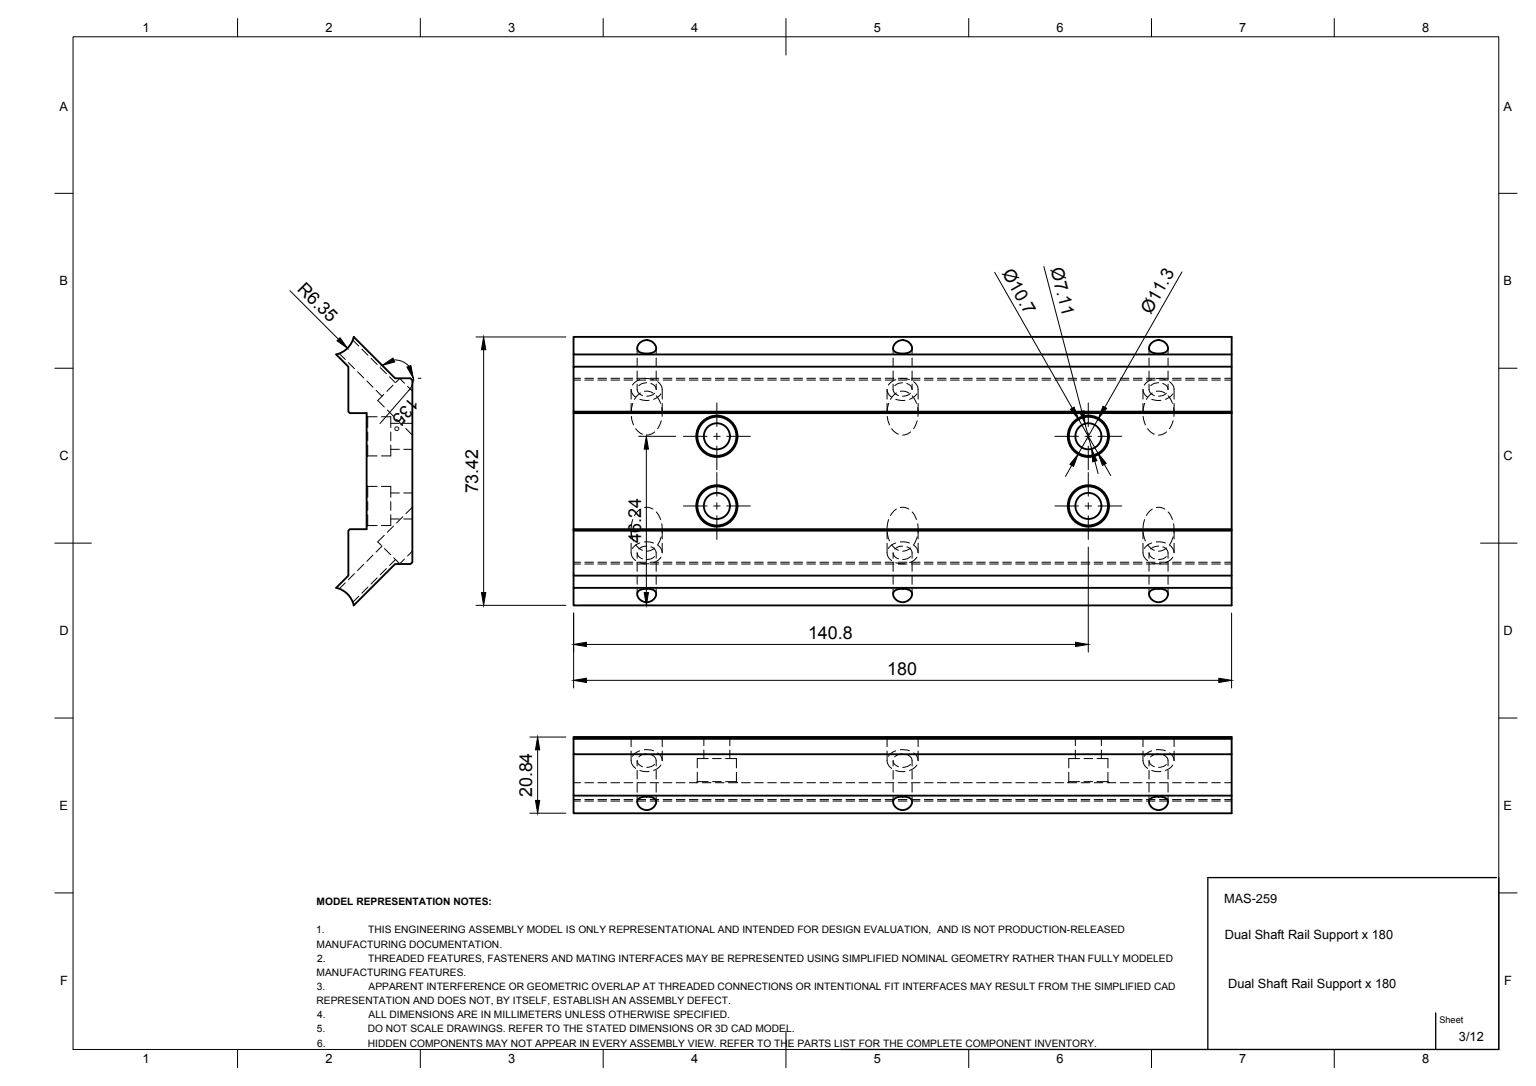
ISO-10303-21;
HEADER;
/* Generated by software containing ST-Developer
 * from STEP Tools, Inc. (www.steptools.com) 
 */

FILE_DESCRIPTION(
/* description */ (''),
/* implementation_level */ '2;1');

FILE_NAME(
/* name */ 'Dual Shaft Rail Support x 180.step',
/* time_stamp */ '2026-10-15T13:30:17-07:00',
/* author */ (''),
/* organization */ (''),
/* preprocessor_version */ 'ST-DEVELOPER v20.2',
/* originating_system */ 'Autodesk Translation Framework v15.15.0.0',
/* authorisation */ '');

FILE_SCHEMA (('AUTOMOTIVE_DESIGN { 1 0 10303 214 3 1 1 }'));
ENDSEC;

DATA;
#10=MECHANICAL_DESIGN_GEOMETRIC_PRESENTATION_REPRESENTATION('',(#1033),#71795);
#1013=SHAPE_REPRESENTATION_RELATIONSHIP('SRR','None',#72017,#1023);
#1023=ADVANCED_BREP_SHAPE_REPRESENTATION('',(#1043),#71785);
#1033=STYLED_ITEM('',(#72076),#1043);
#1043=MANIFOLD_SOLID_BREP('Body1',#13635);
#1053=CONICAL_SURFACE('',#13794,5.5,0.785398163397437);
#1054=CONICAL_SURFACE('',#13803,5.5,0.785398163397452);
#1055=CONICAL_SURFACE('',#13807,5.5,0.785398163397452);
#1056=CONICAL_SURFACE('',#13811,5.5,0.785398163397437);
#1103=B_SPLINE_CURVE_WITH_KNOTS('',3,(#18543,#18544,#18545,#18546,#18547,
#18548,#18549,#18550,#18551,#18552,#18553,#18554,#18555,#18556,#18557,#18558,
#18559,#18560),.UNSPECIFIED.,.F.,.F.,(4,2,2,2,2,2,2,2,4),(-1.58749465662543,
-1.48822066272646,-1.3889466688275,-1.28978383064828,-1.19062099246907,
-1.09145815428986,-0.992295316110649,-0.893021322211684,-0.793747328312718),
 .UNSPECIFIED.);
#1104=B_SPLINE_CURVE_WITH_KNOTS('',3,(#18561,#18562,#18563,#18564,#18565,
#18566,#18567,#18568,#18569,#18570,#18571,#18572,#18573,#18574,#18575,#18576,
#18577,#18578),.UNSPECIFIED.,.F.,.F.,(4,2,2,2,2,2,2,2,4),(-0.793747328312718,
-0.694473334413751,-0.595199340514785,-0.496036502335572,-0.39687366415636,
-0.297710825977147,-0.198547987797934,-0.0992739938989668,0.),
 .UNSPECIFIED.);
#1105=B_SPLINE_CURVE_WITH_KNOTS('',3,(#18592,#18593,#18594,#18595,#18596,
#18597,#18598,#18599,#18600,#18601,#18602,#18603,#18604,#18605,#18606,#18607,
#18608,#18609),.UNSPECIFIED.,.F.,.F.,(4,2,2,2,2,2,2,2,4),(-1.58749465662543,
-1.48822066272646,-1.38894666882749,-1.28978383064828,-1.19062099246907,
-1.09145815428986,-0.992295316110645,-0.893021322211679,-0.793747328312713),
 .UNSPECIFIED.);
#1106=B_SPLINE_CURVE_WITH_KNOTS('',3,(#18610,#18611,#18612,#18613,#18614,
#18615,#18616,#18617,#18618,#18619,#18620,#18621,#18622,#18623,#18624,#18625,
#18626,#18627),.UNSPECIFIED.,.F.,.F.,(4,2,2,2,2,2,2,2,4),(-0.793747328312713,
-0.694473334413747,-0.595199340514781,-0.496036502335569,-0.396873664156357,
-0.297710825977144,-0.198547987797932,-0.0992739938989662,0.),
 .UNSPECIFIED.);
#1107=B_SPLINE_CURVE_WITH_KNOTS('',3,(#18641,#18642,#18643,#18644,#18645,
#18646,#18647,#18648,#18649,#18650,#18651,#18652,#18653,#18654,#18655,#18656,
#18657,#18658),.UNSPECIFIED.,.F.,.F.,(4,2,2,2,2,2,2,2,4),(-1.58749465662542,
-1.48822066272646,-1.38894666882749,-1.28978383064828,-1.19062099246907,
-1.09145815428986,-0.992295316110644,-0.893021322211679,-0.793747328312713),
 .UNSPECIFIED.);
#1108=B_SPLINE_CURVE_WITH_KNOTS('',3,(#18659,#18660,#18661,#18662,#18663,
#18664,#18665,#18666,#18667,#18668,#18669,#18670,#18671,#18672,#18673,#18674,
#18675,#18676),.UNSPECIFIED.,.F.,.F.,(4,2,2,2,2,2,2,2,4),(-0.793747328312713,
-0.694473334413747,-0.595199340514781,-0.496036502335569,-0.396873664156357,
-0.297710825977144,-0.198547987797932,-0.099273993898966,0.),
 .UNSPECIFIED.);
#1109=B_SPLINE_CURVE_WITH_KNOTS('',3,(#18690,#18691,#18692,#18693,#18694,
#18695,#18696,#18697,#18698,#18699,#18700,#18701,#18702,#18703,#18704,#18705,
#18706,#18707),.UNSPECIFIED.,.F.,.F.,(4,2,2,2,2,2,2,2,4),(-1.58749465662543,
-1.48822066272646,-1.3889466688275,-1.28978383064828,-1.19062099246907,
-1.09145815428986,-0.992295316110649,-0.893021322211684,-0.793747328312718),
 .UNSPECIFIED.);
#1110=B_SPLINE_CURVE_WITH_KNOTS('',3,(#18708,#18709,#18710,#18711,#18712,
#18713,#18714,#18715,#18716,#18717,#18718,#18719,#18720,#18721,#18722,#18723,
#18724,#18725),.UNSPECIFIED.,.F.,.F.,(4,2,2,2,2,2,2,2,4),(-0.793747328312718,
-0.694473334413751,-0.595199340514785,-0.496036502335572,-0.396873664156359,
-0.297710825977146,-0.198547987797934,-0.0992739938989669,0.),
 .UNSPECIFIED.);
#1111=B_SPLINE_CURVE_WITH_KNOTS('',3,(#18739,#18740,#18741,#18742,#18743,
#18744,#18745,#18746,#18747,#18748,#18749,#18750,#18751,#18752,#18753,#18754,
#18755,#18756),.UNSPECIFIED.,.F.,.F.,(4,2,2,2,2,2,2,2,4),(-1.58749465662543,
-1.48822066272646,-1.38894666882749,-1.28978383064828,-1.19062099246907,
-1.09145815428986,-0.992295316110645,-0.893021322211679,-0.793747328312713),
 .UNSPECIFIED.);
#1112=B_SPLINE_CURVE_WITH_KNOTS('',3,(#18757,#18758,#18759,#18760,#18761,
#18762,#18763,#18764,#18765,#18766,#18767,#18768,#18769,#18770,#18771,#18772,
#18773,#18774),.UNSPECIFIED.,.F.,.F.,(4,2,2,2,2,2,2,2,4),(-0.793747328312713,
-0.694473334413747,-0.595199340514781,-0.496036502335568,-0.396873664156356,
-0.297710825977144,-0.198547987797932,-0.099273993898966,0.),
 .UNSPECIFIED.);
#1113=B_SPLINE_CURVE_WITH_KNOTS('',3,(#18788,#18789,#18790,#18791,#18792,
#18793,#18794,#18795,#18796,#18797,#18798,#18799,#18800,#18801,#18802,#18803,
#18804,#18805),.UNSPECIFIED.,.F.,.F.,(4,2,2,2,2,2,2,2,4),(-1.58749465662543,
-1.48822066272646,-1.38894666882749,-1.28978383064828,-1.19062099246907,
-1.09145815428986,-0.992295316110644,-0.893021322211679,-0.793747328312713),
 .UNSPECIFIED.);
#1114=B_SPLINE_CURVE_WITH_KNOTS('',3,(#18806,#18807,#18808,#18809,#18810,
#18811,#18812,#18813,#18814,#18815,#18816,#18817,#18818,#18819,#18820,#18821,
#18822,#18823),.UNSPECIFIED.,.F.,.F.,(4,2,2,2,2,2,2,2,4),(-0.793747328312713,
-0.694473334413747,-0.595199340514781,-0.496036502335569,-0.396873664156356,
-0.297710825977144,-0.198547987797932,-0.0992739938989659,0.),
 .UNSPECIFIED.);
#1484=FACE_BOUND('',#2677,.T.);
#1485=FACE_BOUND('',#2681,.T.);
#1486=FACE_BOUND('',#2685,.T.);
#1487=FACE_BOUND('',#2689,.T.);
#1488=FACE_BOUND('',#2693,.T.);
#1489=FACE_BOUND('',#2697,.T.);
#1490=FACE_BOUND('',#2701,.T.);
#1491=FACE_BOUND('',#2702,.T.);
#1492=FACE_BOUND('',#2703,.T.);
#1493=FACE_BOUND('',#2704,.T.);
#1494=FACE_BOUND('',#2713,.T.);
#1495=FACE_BOUND('',#2715,.T.);
#1496=FACE_BOUND('',#2717,.T.);
#1497=FACE_BOUND('',#2719,.T.);
#1498=FACE_BOUND('',#2731,.T.);
#1499=FACE_BOUND('',#2732,.T.);
#1500=FACE_BOUND('',#2733,.T.);
#1501=FACE_BOUND('',#2734,.T.);
#1502=FACE_BOUND('',#2735,.T.);
#1503=FACE_BOUND('',#2736,.T.);
#1504=FACE_BOUND('',#2737,.T.);
#1505=FACE_BOUND('',#2738,.T.);
#1506=FACE_BOUND('',#2739,.T.);
#1507=FACE_BOUND('',#2740,.T.);
#1508=FACE_BOUND('',#2743,.T.);
#1509=FACE_BOUND('',#2744,.T.);
#1510=FACE_BOUND('',#2745,.T.);
#1511=FACE_BOUND('',#2751,.T.);
#1512=FACE_BOUND('',#2752,.T.);
#1513=FACE_BOUND('',#2753,.T.);
#1565=PLANE('',#13761);
#1566=PLANE('',#13767);
#1567=PLANE('',#13773);
#1568=PLANE('',#13779);
#1569=PLANE('',#13785);
#1570=PLANE('',#13791);
#1571=PLANE('',#13797);
#1572=PLANE('',#13815);
#1573=PLANE('',#13817);
#1574=PLANE('',#13819);
#1575=PLANE('',#13821);
#1576=PLANE('',#13831);
#1577=PLANE('',#13832);
#1578=PLANE('',#13833);
#1579=PLANE('',#13836);
#1580=PLANE('',#13837);
#1581=PLANE('',#13838);
#1582=PLANE('',#13839);
#1583=PLANE('',#13840);
#1584=PLANE('',#13843);
#1585=PLANE('',#13844);
#1586=PLANE('',#13845);
#1587=PLANE('',#13846);
#1588=PLANE('',#13849);
#1589=PLANE('',#13850);
#1590=PLANE('',#13851);
#1591=PLANE('',#13852);
#1592=PLANE('',#13853);
#2027=FACE_OUTER_BOUND('',#2675,.T.);
#2028=FACE_OUTER_BOUND('',#2676,.T.);
#2029=FACE_OUTER_BOUND('',#2678,.T.);
#2030=FACE_OUTER_BOUND('',#2679,.T.);
#2031=FACE_OUTER_BOUND('',#2680,.T.);
#2032=FACE_OUTER_BOUND('',#2682,.T.);
#2033=FACE_OUTER_BOUND('',#2683,.T.);
#2034=FACE_OUTER_BOUND('',#2684,.T.);
#2035=FACE_OUTER_BOUND('',#2686,.T.);
#2036=FACE_OUTER_BOUND('',#2687,.T.);
#2037=FACE_OUTER_BOUND('',#2688,.T.);
#2038=FACE_OUTER_BOUND('',#2690,.T.);
#2039=FACE_OUTER_BOUND('',#2691,.T.);
#2040=FACE_OUTER_BOUND('',#2692,.T.);
#2041=FACE_OUTER_BOUND('',#2694,.T.);
#2042=FACE_OUTER_BOUND('',#2695,.T.);
#2043=FACE_OUTER_BOUND('',#2696,.T.);
#2044=FACE_OUTER_BOUND('',#2698,.T.);
#2045=FACE_OUTER_BOUND('',#2699,.T.);
#2046=FACE_OUTER_BOUND('',#2700,.T.);
#2047=FACE_OUTER_BOUND('',#2705,.T.);
#2048=FACE_OUTER_BOUND('',#2706,.T.);
#2049=FACE_OUTER_BOUND('',#2707,.T.);
#2050=FACE_OUTER_BOUND('',#2708,.T.);
#2051=FACE_OUTER_BOUND('',#2709,.T.);
#2052=FACE_OUTER_BOUND('',#2710,.T.);
#2053=FACE_OUTER_BOUND('',#2711,.T.);
#2054=FACE_OUTER_BOUND('',#2712,.T.);
#2055=FACE_OUTER_BOUND('',#2714,.T.);
#2056=FACE_OUTER_BOUND('',#2716,.T.);
#2057=FACE_OUTER_BOUND('',#2718,.T.);
#2058=FACE_OUTER_BOUND('',#2720,.T.);
#2059=FACE_OUTER_BOUND('',#2721,.T.);
#2060=FACE_OUTER_BOUND('',#2722,.T.);
#2061=FACE_OUTER_BOUND('',#2723,.T.);
#2062=FACE_OUTER_BOUND('',#2724,.T.);
#2063=FACE_OUTER_BOUND('',#2725,.T.);
#2064=FACE_OUTER_BOUND('',#2726,.T.);
#2065=FACE_OUTER_BOUND('',#2727,.T.);
#2066=FACE_OUTER_BOUND('',#2728,.T.);
#2067=FACE_OUTER_BOUND('',#2729,.T.);
#2068=FACE_OUTER_BOUND('',#2730,.T.);
#2069=FACE_OUTER_BOUND('',#2741,.T.);
#2070=FACE_OUTER_BOUND('',#2742,.T.);
#2071=FACE_OUTER_BOUND('',#2746,.T.);
#2072=FACE_OUTER_BOUND('',#2747,.T.);
#2073=FACE_OUTER_BOUND('',#2748,.T.);
#2074=FACE_OUTER_BOUND('',#2749,.T.);
#2075=FACE_OUTER_BOUND('',#2750,.T.);
#2076=FACE_OUTER_BOUND('',#2754,.T.);
#2077=FACE_OUTER_BOUND('',#2755,.T.);
#2078=FACE_OUTER_BOUND('',#2756,.T.);
#2079=FACE_OUTER_BOUND('',#2757,.T.);
#2080=FACE_OUTER_BOUND('',#2758,.T.);
#2675=EDGE_LOOP('',(#8965,#8966,#8967,#8968));
#2676=EDGE_LOOP('',(#8969));
#2677=EDGE_LOOP('',(#8970));
#2678=EDGE_LOOP('',(#8971,#8972,#8973,#8974,#8975));
#2679=EDGE_LOOP('',(#8976,#8977,#8978,#8979));
#2680=EDGE_LOOP('',(#8980));
#2681=EDGE_LOOP('',(#8981));
#2682=EDGE_LOOP('',(#8982,#8983,#8984,#8985,#8986));
#2683=EDGE_LOOP('',(#8987,#8988,#8989,#8990));
#2684=EDGE_LOOP('',(#8991));
#2685=EDGE_LOOP('',(#8992));
#2686=EDGE_LOOP('',(#8993,#8994,#8995,#8996,#8997));
#2687=EDGE_LOOP('',(#8998,#8999,#9000,#9001));
#2688=EDGE_LOOP('',(#9002));
#2689=EDGE_LOOP('',(#9003));
#2690=EDGE_LOOP('',(#9004,#9005,#9006,#9007,#9008));
#2691=EDGE_LOOP('',(#9009,#9010,#9011,#9012));
#2692=EDGE_LOOP('',(#9013));
#2693=EDGE_LOOP('',(#9014));
#2694=EDGE_LOOP('',(#9015,#9016,#9017,#9018,#9019));
#2695=EDGE_LOOP('',(#9020,#9021,#9022,#9023));
#2696=EDGE_LOOP('',(#9024));
#2697=EDGE_LOOP('',(#9025));
#2698=EDGE_LOOP('',(#9026,#9027,#9028,#9029,#9030));
#2699=EDGE_LOOP('',(#9031,#9032,#9033,#9034));
#2700=EDGE_LOOP('',(#9035,#9036,#9037,#9038));
#2701=EDGE_LOOP('',(#9039));
#2702=EDGE_LOOP('',(#9040));
#2703=EDGE_LOOP('',(#9041));
#2704=EDGE_LOOP('',(#9042));
#2705=EDGE_LOOP('',(#9043,#9044,#9045,#9046));
#2706=EDGE_LOOP('',(#9047,#9048,#9049,#9050));
#2707=EDGE_LOOP('',(#9051,#9052,#9053,#9054));
#2708=EDGE_LOOP('',(#9055,#9056,#9057,#9058));
#2709=EDGE_LOOP('',(#9059,#9060,#9061,#9062));
#2710=EDGE_LOOP('',(#9063,#9064,#9065,#9066));
#2711=EDGE_LOOP('',(#9067,#9068,#9069,#9070));
#2712=EDGE_LOOP('',(#9071));
#2713=EDGE_LOOP('',(#9072));
#2714=EDGE_LOOP('',(#9073));
#2715=EDGE_LOOP('',(#9074));
#2716=EDGE_LOOP('',(#9075));
#2717=EDGE_LOOP('',(#9076));
#2718=EDGE_LOOP('',(#9077));
#2719=EDGE_LOOP('',(#9078));
#2720=EDGE_LOOP('',(#9079,#9080,#9081,#9082));
#2721=EDGE_LOOP('',(#9083,#9084,#9085,#9086));
#2722=EDGE_LOOP('',(#9087,#9088,#9089,#9090));
#2723=EDGE_LOOP('',(#9091,#9092,#9093,#9094));
#2724=EDGE_LOOP('',(#9095,#9096,#9097,#9098));
#2725=EDGE_LOOP('',(#9099,#9100,#9101,#9102));
#2726=EDGE_LOOP('',(#9103,#9104,#9105,#9106,#9107,#9108,#9109,#9110,#9111,
#9112,#9113,#9114,#9115,#9116,#9117,#9118,#9119,#9120));
#2727=EDGE_LOOP('',(#9121,#9122,#9123,#9124));
#2728=EDGE_LOOP('',(#9125,#9126,#9127,#9128));
#2729=EDGE_LOOP('',(#9129,#9130,#9131,#9132));
#2730=EDGE_LOOP('',(#9133,#9134,#9135,#9136));
#2731=EDGE_LOOP('',(#9137));
#2732=EDGE_LOOP('',(#9138));
#2733=EDGE_LOOP('',(#9139));
#2734=EDGE_LOOP('',(#9140));
#2735=EDGE_LOOP('',(#9141));
#2736=EDGE_LOOP('',(#9142));
#2737=EDGE_LOOP('',(#9143));
#2738=EDGE_LOOP('',(#9144));
#2739=EDGE_LOOP('',(#9145));
#2740=EDGE_LOOP('',(#9146));
#2741=EDGE_LOOP('',(#9147,#9148,#9149,#9150));
#2742=EDGE_LOOP('',(#9151,#9152,#9153,#9154));
#2743=EDGE_LOOP('',(#9155,#9156));
#2744=EDGE_LOOP('',(#9157,#9158));
#2745=EDGE_LOOP('',(#9159,#9160));
#2746=EDGE_LOOP('',(#9161,#9162,#9163,#9164));
#2747=EDGE_LOOP('',(#9165,#9166,#9167,#9168));
#2748=EDGE_LOOP('',(#9169,#9170,#9171,#9172));
#2749=EDGE_LOOP('',(#9173,#9174,#9175,#9176));
#2750=EDGE_LOOP('',(#9177,#9178,#9179,#9180));
#2751=EDGE_LOOP('',(#9181,#9182));
#2752=EDGE_LOOP('',(#9183,#9184));
#2753=EDGE_LOOP('',(#9185,#9186));
#2754=EDGE_LOOP('',(#9187,#9188,#9189,#9190));
#2755=EDGE_LOOP('',(#9191,#9192,#9193,#9194));
#2756=EDGE_LOOP('',(#9195,#9196,#9197,#9198));
#2757=EDGE_LOOP('',(#9199,#9200,#9201,#9202));
#2758=EDGE_LOOP('',(#9203,#9204,#9205,#9206,#9207,#9208,#9209,#9210,#9211,
#9212,#9213,#9214,#9215,#9216,#9217,#9218,#9219,#9220));
#3404=CIRCLE('',#13760,4.25);
#3405=CIRCLE('',#13762,2.6);
#3406=CIRCLE('',#13766,4.25);
#3407=CIRCLE('',#13768,2.6);
#3408=CIRCLE('',#13772,4.25);
#3409=CIRCLE('',#13774,2.6);
#3410=CIRCLE('',#13778,4.25);
#3411=CIRCLE('',#13780,2.6);
#3412=CIRCLE('',#13784,4.25);
#3413=CIRCLE('',#13786,2.6);
#3414=CIRCLE('',#13790,4.25);
#3415=CIRCLE('',#13792,2.6);
#3416=CIRCLE('',#13795,5.35);
#3417=CIRCLE('',#13796,5.65);
#3418=CIRCLE('',#13798,5.65);
#3419=CIRCLE('',#13799,5.65);
#3420=CIRCLE('',#13800,5.65);
#3421=CIRCLE('',#13802,5.35);
#3422=CIRCLE('',#13804,5.35);
#3423=CIRCLE('',#13806,5.35);
#3424=CIRCLE('',#13808,5.35);
#3425=CIRCLE('',#13810,5.35);
#3426=CIRCLE('',#13812,5.35);
#3427=CIRCLE('',#13814,5.35);
#3428=CIRCLE('',#13816,3.55600000000001);
#3429=CIRCLE('',#13818,3.556);
#3430=CIRCLE('',#13820,3.556);
#3431=CIRCLE('',#13822,3.55600000000001);
#3432=CIRCLE('',#13824,3.55600000000001);
#3433=CIRCLE('',#13826,3.556);
#3434=CIRCLE('',#13828,3.556);
#3435=CIRCLE('',#13830,3.55600000000001);
#3436=CIRCLE('',#13834,6.35);
#3437=CIRCLE('',#13835,6.35);
#3438=CIRCLE('',#13842,6.35);
#3439=CIRCLE('',#13848,6.35);
#3838=LINE('',#18534,#4749);
#3839=LINE('',#18541,#4750);
#3840=LINE('',#18583,#4751);
#3841=LINE('',#18590,#4752);
#3842=LINE('',#18632,#4753);
#3843=LINE('',#18639,#4754);
#3844=LINE('',#18681,#4755);
#3845=LINE('',#18688,#4756);
#3846=LINE('',#18730,#4757);
#3847=LINE('',#18737,#4758);
#3848=LINE('',#18779,#4759);
#3849=LINE('',#18786,#4760);
#3850=LINE('',#18828,#4761);
#3851=LINE('',#18833,#4762);
#3852=LINE('',#18835,#4763);
#3853=LINE('',#18837,#4764);
#3854=LINE('',#18838,#4765);
#3855=LINE('',#18847,#4766);
#3856=LINE('',#18852,#4767);
#3857=LINE('',#18855,#4768);
#3858=LINE('',#18860,#4769);
#3859=LINE('',#18863,#4770);
#3860=LINE('',#18868,#4771);
#3861=LINE('',#18871,#4772);
#3862=LINE('',#18887,#4773);
#3863=LINE('',#18891,#4774);
#3864=LINE('',#18895,#4775);
#3865=LINE('',#18899,#4776);
#3866=LINE('',#18904,#4777);
#3867=LINE('',#18906,#4778);
#3868=LINE('',#18908,#4779);
#3869=LINE('',#18909,#4780);
#3870=LINE('',#18911,#4781);
#3871=LINE('',#18912,#4782);
#3872=LINE('',#18915,#4783);
#3873=LINE('',#18917,#4784);
#3874=LINE('',#18921,#4785);
#3875=LINE('',#18923,#4786);
#3876=LINE('',#18925,#4787);
#3877=LINE('',#18927,#4788);
#3878=LINE('',#18929,#4789);
#3879=LINE('',#18931,#4790);
#3880=LINE('',#18933,#4791);
#3881=LINE('',#18937,#4792);
#3882=LINE('',#18939,#4793);
#3883=LINE('',#18941,#4794);
#3884=LINE('',#18942,#4795);
#3885=LINE('',#18946,#4796);
#3886=LINE('',#18947,#4797);
#3887=LINE('',#18948,#4798);
#3888=LINE('',#18951,#4799);
#3889=LINE('',#18952,#4800);
#3890=LINE('',#18956,#4801);
#3891=LINE('',#18957,#4802);
#3892=LINE('',#18958,#4803);
#3893=LINE('',#18961,#4804);
#3894=LINE('',#18962,#4805);
#3895=LINE('',#18965,#4806);
#3896=LINE('',#18966,#4807);
#3897=LINE('',#18969,#4808);
#3898=LINE('',#18972,#4809);
#3899=LINE('',#18975,#4810);
#3900=LINE('',#18976,#4811);
#3901=LINE('',#18978,#4812);
#3902=LINE('',#18981,#4813);
#3903=LINE('',#18982,#4814);
#3904=LINE('',#18985,#4815);
#3905=LINE('',#18986,#4816);
#3906=LINE('',#18990,#4817);
#3907=LINE('',#18992,#4818);
#3908=LINE('',#18994,#4819);
#3909=LINE('',#18997,#4820);
#3910=LINE('',#18998,#4821);
#3911=LINE('',#19000,#4822);
#4749=VECTOR('',#15051,4.25);
#4750=VECTOR('',#15060,2.6);
#4751=VECTOR('',#15065,4.25);
#4752=VECTOR('',#15074,2.6);
#4753=VECTOR('',#15079,4.25);
#4754=VECTOR('',#15088,2.6);
#4755=VECTOR('',#15093,4.25);
#4756=VECTOR('',#15102,2.6);
#4757=VECTOR('',#15107,4.25);
#4758=VECTOR('',#15116,2.6);
#4759=VECTOR('',#15121,4.25);
#4760=VECTOR('',#15130,2.6);
#4761=VECTOR('',#15135,5.5);
#4762=VECTOR('',#15140,10.);
#4763=VECTOR('',#15141,10.);
#4764=VECTOR('',#15142,10.);
#4765=VECTOR('',#15143,10.);
#4766=VECTOR('',#15152,5.35);
#4767=VECTOR('',#15159,5.5);
#4768=VECTOR('',#15162,5.35);
#4769=VECTOR('',#15169,5.5);
#4770=VECTOR('',#15172,5.35);
#4771=VECTOR('',#15179,5.5);
#4772=VECTOR('',#15182,5.35);
#4773=VECTOR('',#15203,3.55600000000001);
#4774=VECTOR('',#15208,3.556);
#4775=VECTOR('',#15213,3.556);
#4776=VECTOR('',#15218,3.55600000000001);
#4777=VECTOR('',#15223,10.);
#4778=VECTOR('',#15224,10.);
#4779=VECTOR('',#15225,10.);
#4780=VECTOR('',#15226,10.);
#4781=VECTOR('',#15229,10.);
#4782=VECTOR('',#15230,10.);
#4783=VECTOR('',#15233,10.);
#4784=VECTOR('',#15234,10.);
#4785=VECTOR('',#15237,10.);
#4786=VECTOR('',#15238,10.);
#4787=VECTOR('',#15239,10.);
#4788=VECTOR('',#15240,10.);
#4789=VECTOR('',#15241,10.);
#4790=VECTOR('',#15242,10.);
#4791=VECTOR('',#15243,10.);
#4792=VECTOR('',#15246,10.);
#4793=VECTOR('',#15247,10.);
#4794=VECTOR('',#15248,10.);
#4795=VECTOR('',#15249,10.);
#4796=VECTOR('',#15252,10.);
#4797=VECTOR('',#15253,10.);
#4798=VECTOR('',#15254,10.);
#4799=VECTOR('',#15257,10.);
#4800=VECTOR('',#15258,10.);
#4801=VECTOR('',#15261,10.);
#4802=VECTOR('',#15262,10.);
#4803=VECTOR('',#15263,10.);
#4804=VECTOR('',#15266,10.);
#4805=VECTOR('',#15267,10.);
#4806=VECTOR('',#15270,10.);
#4807=VECTOR('',#15271,10.);
#4808=VECTOR('',#15274,10.);
#4809=VECTOR('',#15277,10.);
#4810=VECTOR('',#15280,10.);
#4811=VECTOR('',#15281,10.);
#4812=VECTOR('',#15284,10.);
#4813=VECTOR('',#15287,10.);
#4814=VECTOR('',#15288,10.);
#4815=VECTOR('',#15291,10.);
#4816=VECTOR('',#15292,10.);
#4817=VECTOR('',#15297,10.);
#4818=VECTOR('',#15300,10.);
#4819=VECTOR('',#15303,10.);
#4820=VECTOR('',#15306,10.);
#4821=VECTOR('',#15307,10.);
#4822=VECTOR('',#15310,10.);
#5660=ELLIPSE('',#13759,6.01040764008565,4.25);
#5661=ELLIPSE('',#13765,6.01040764008565,4.25);
#5662=ELLIPSE('',#13771,6.01040764008565,4.25);
#5663=ELLIPSE('',#13777,6.01040764008566,4.25);
#5664=ELLIPSE('',#13783,6.01040764008566,4.25);
#5665=ELLIPSE('',#13789,6.01040764008566,4.25);
#5666=VERTEX_POINT('',#18531);
#5667=VERTEX_POINT('',#18533);
#5668=VERTEX_POINT('',#18537);
#5669=VERTEX_POINT('',#18540);
#5670=VERTEX_POINT('',#18542);
#5671=VERTEX_POINT('',#18580);
#5672=VERTEX_POINT('',#18582);
#5673=VERTEX_POINT('',#18586);
#5674=VERTEX_POINT('',#18589);
#5675=VERTEX_POINT('',#18591);
#5676=VERTEX_POINT('',#18629);
#5677=VERTEX_POINT('',#18631);
#5678=VERTEX_POINT('',#18635);
#5679=VERTEX_POINT('',#18638);
#5680=VERTEX_POINT('',#18640);
#5681=VERTEX_POINT('',#18678);
#5682=VERTEX_POINT('',#18680);
#5683=VERTEX_POINT('',#18684);
#5684=VERTEX_POINT('',#18687);
#5685=VERTEX_POINT('',#18689);
#5686=VERTEX_POINT('',#18727);
#5687=VERTEX_POINT('',#18729);
#5688=VERTEX_POINT('',#18733);
#5689=VERTEX_POINT('',#18736);
#5690=VERTEX_POINT('',#18738);
#5691=VERTEX_POINT('',#18776);
#5692=VERTEX_POINT('',#18778);
#5693=VERTEX_POINT('',#18782);
#5694=VERTEX_POINT('',#18785);
#5695=VERTEX_POINT('',#18787);
#5696=VERTEX_POINT('',#18825);
#5697=VERTEX_POINT('',#18827);
#5698=VERTEX_POINT('',#18831);
#5699=VERTEX_POINT('',#18832);
#5700=VERTEX_POINT('',#18834);
#5701=VERTEX_POINT('',#18836);
#5702=VERTEX_POINT('',#18839);
#5703=VERTEX_POINT('',#18841);
#5704=VERTEX_POINT('',#18843);
#5705=VERTEX_POINT('',#18846);
#5706=VERTEX_POINT('',#18850);
#5707=VERTEX_POINT('',#18854);
#5708=VERTEX_POINT('',#18858);
#5709=VERTEX_POINT('',#18862);
#5710=VERTEX_POINT('',#18866);
#5711=VERTEX_POINT('',#18870);
#5712=VERTEX_POINT('',#18874);
#5713=VERTEX_POINT('',#18877);
#5714=VERTEX_POINT('',#18880);
#5715=VERTEX_POINT('',#18883);
#5716=VERTEX_POINT('',#18886);
#5717=VERTEX_POINT('',#18890);
#5718=VERTEX_POINT('',#18894);
#5719=VERTEX_POINT('',#18898);
#5720=VERTEX_POINT('',#18902);
#5721=VERTEX_POINT('',#18903);
#5722=VERTEX_POINT('',#18905);
#5723=VERTEX_POINT('',#18907);
#5724=VERTEX_POINT('',#18914);
#5725=VERTEX_POINT('',#18916);
#5726=VERTEX_POINT('',#18918);
#5727=VERTEX_POINT('',#18920);
#5728=VERTEX_POINT('',#18922);
#5729=VERTEX_POINT('',#18924);
#5730=VERTEX_POINT('',#18926);
#5731=VERTEX_POINT('',#18928);
#5732=VERTEX_POINT('',#18930);
#5733=VERTEX_POINT('',#18932);
#5734=VERTEX_POINT('',#18934);
#5735=VERTEX_POINT('',#18936);
#5736=VERTEX_POINT('',#18938);
#5737=VERTEX_POINT('',#18940);
#5738=VERTEX_POINT('',#18944);
#5739=VERTEX_POINT('',#18945);
#5740=VERTEX_POINT('',#18950);
#5741=VERTEX_POINT('',#18954);
#5742=VERTEX_POINT('',#18955);
#5743=VERTEX_POINT('',#18960);
#5744=VERTEX_POINT('',#18964);
#5745=VERTEX_POINT('',#18968);
#5746=VERTEX_POINT('',#18970);
#5747=VERTEX_POINT('',#18974);
#5748=VERTEX_POINT('',#18980);
#5749=VERTEX_POINT('',#18984);
#5750=VERTEX_POINT('',#18988);
#5751=VERTEX_POINT('',#18996);
#7017=EDGE_CURVE('',#5666,#5666,#5660,.T.);
#7018=EDGE_CURVE('',#5666,#5667,#3838,.T.);
#7019=EDGE_CURVE('',#5667,#5667,#3404,.T.);
#7020=EDGE_CURVE('',#5668,#5668,#3405,.T.);
#7021=EDGE_CURVE('',#5668,#5669,#3839,.T.);
#7022=EDGE_CURVE('',#5670,#5669,#1103,.T.);
#7023=EDGE_CURVE('',#5669,#5670,#1104,.T.);
#7024=EDGE_CURVE('',#5671,#5671,#5661,.T.);
#7025=EDGE_CURVE('',#5671,#5672,#3840,.T.);
#7026=EDGE_CURVE('',#5672,#5672,#3406,.T.);
#7027=EDGE_CURVE('',#5673,#5673,#3407,.T.);
#7028=EDGE_CURVE('',#5673,#5674,#3841,.T.);
#7029=EDGE_CURVE('',#5675,#5674,#1105,.T.);
#7030=EDGE_CURVE('',#5674,#5675,#1106,.T.);
#7031=EDGE_CURVE('',#5676,#5676,#5662,.T.);
#7032=EDGE_CURVE('',#5676,#5677,#3842,.T.);
#7033=EDGE_CURVE('',#5677,#5677,#3408,.T.);
#7034=EDGE_CURVE('',#5678,#5678,#3409,.T.);
#7035=EDGE_CURVE('',#5678,#5679,#3843,.T.);
#7036=EDGE_CURVE('',#5680,#5679,#1107,.T.);
#7037=EDGE_CURVE('',#5679,#5680,#1108,.T.);
#7038=EDGE_CURVE('',#5681,#5681,#5663,.T.);
#7039=EDGE_CURVE('',#5681,#5682,#3844,.T.);
#7040=EDGE_CURVE('',#5682,#5682,#3410,.T.);
#7041=EDGE_CURVE('',#5683,#5683,#3411,.T.);
#7042=EDGE_CURVE('',#5683,#5684,#3845,.T.);
#7043=EDGE_CURVE('',#5685,#5684,#1109,.T.);
#7044=EDGE_CURVE('',#5684,#5685,#1110,.T.);
#7045=EDGE_CURVE('',#5686,#5686,#5664,.T.);
#7046=EDGE_CURVE('',#5686,#5687,#3846,.T.);
#7047=EDGE_CURVE('',#5687,#5687,#3412,.T.);
#7048=EDGE_CURVE('',#5688,#5688,#3413,.T.);
#7049=EDGE_CURVE('',#5688,#5689,#3847,.T.);
#7050=EDGE_CURVE('',#5690,#5689,#1111,.T.);
#7051=EDGE_CURVE('',#5689,#5690,#1112,.T.);
#7052=EDGE_CURVE('',#5691,#5691,#5665,.T.);
#7053=EDGE_CURVE('',#5691,#5692,#3848,.T.);
#7054=EDGE_CURVE('',#5692,#5692,#3414,.T.);
#7055=EDGE_CURVE('',#5693,#5693,#3415,.T.);
#7056=EDGE_CURVE('',#5693,#5694,#3849,.T.);
#7057=EDGE_CURVE('',#5695,#5694,#1113,.T.);
#7058=EDGE_CURVE('',#5694,#5695,#1114,.T.);
#7059=EDGE_CURVE('',#5696,#5696,#3416,.T.);
#7060=EDGE_CURVE('',#5696,#5697,#3850,.T.);
#7061=EDGE_CURVE('',#5697,#5697,#3417,.T.);
#7062=EDGE_CURVE('',#5698,#5699,#3851,.T.);
#7063=EDGE_CURVE('',#5699,#5700,#3852,.T.);
#7064=EDGE_CURVE('',#5701,#5700,#3853,.T.);
#7065=EDGE_CURVE('',#5698,#5701,#3854,.T.);
#7066=EDGE_CURVE('',#5702,#5702,#3418,.T.);
#7067=EDGE_CURVE('',#5703,#5703,#3419,.T.);
#7068=EDGE_CURVE('',#5704,#5704,#3420,.T.);
#7069=EDGE_CURVE('',#5696,#5705,#3855,.T.);
#7070=EDGE_CURVE('',#5705,#5705,#3421,.T.);
#7071=EDGE_CURVE('',#5706,#5706,#3422,.T.);
#7072=EDGE_CURVE('',#5706,#5702,#3856,.T.);
#7073=EDGE_CURVE('',#5706,#5707,#3857,.T.);
#7074=EDGE_CURVE('',#5707,#5707,#3423,.T.);
#7075=EDGE_CURVE('',#5708,#5708,#3424,.T.);
#7076=EDGE_CURVE('',#5708,#5704,#3858,.T.);
#7077=EDGE_CURVE('',#5708,#5709,#3859,.T.);
#7078=EDGE_CURVE('',#5709,#5709,#3425,.T.);
#7079=EDGE_CURVE('',#5710,#5710,#3426,.T.);
#7080=EDGE_CURVE('',#5710,#5703,#3860,.T.);
#7081=EDGE_CURVE('',#5710,#5711,#3861,.T.);
#7082=EDGE_CURVE('',#5711,#5711,#3427,.T.);
#7083=EDGE_CURVE('',#5712,#5712,#3428,.T.);
#7084=EDGE_CURVE('',#5713,#5713,#3429,.T.);
#7085=EDGE_CURVE('',#5714,#5714,#3430,.T.);
#7086=EDGE_CURVE('',#5715,#5715,#3431,.T.);
#7087=EDGE_CURVE('',#5712,#5716,#3862,.T.);
#7088=EDGE_CURVE('',#5716,#5716,#3432,.T.);
#7089=EDGE_CURVE('',#5713,#5717,#3863,.T.);
#7090=EDGE_CURVE('',#5717,#5717,#3433,.T.);
#7091=EDGE_CURVE('',#5714,#5718,#3864,.T.);
#7092=EDGE_CURVE('',#5718,#5718,#3434,.T.);
#7093=EDGE_CURVE('',#5715,#5719,#3865,.T.);
#7094=EDGE_CURVE('',#5719,#5719,#3435,.T.);
#7095=EDGE_CURVE('',#5720,#5721,#3866,.T.);
#7096=EDGE_CURVE('',#5721,#5722,#3867,.T.);
#7097=EDGE_CURVE('',#5722,#5723,#3868,.T.);
#7098=EDGE_CURVE('',#5723,#5720,#3869,.T.);
#7099=EDGE_CURVE('',#5723,#5698,#3870,.T.);
#7100=EDGE_CURVE('',#5720,#5701,#3871,.T.);
#7101=EDGE_CURVE('',#5724,#5722,#3872,.T.);
#7102=EDGE_CURVE('',#5725,#5724,#3873,.T.);
#7103=EDGE_CURVE('',#5725,#5726,#3436,.T.);
#7104=EDGE_CURVE('',#5727,#5726,#3874,.T.);
#7105=EDGE_CURVE('',#5728,#5727,#3875,.T.);
#7106=EDGE_CURVE('',#5729,#5728,#3876,.T.);
#7107=EDGE_CURVE('',#5729,#5730,#3877,.T.);
#7108=EDGE_CURVE('',#5731,#5730,#3878,.T.);
#7109=EDGE_CURVE('',#5731,#5732,#3879,.T.);
#7110=EDGE_CURVE('',#5732,#5733,#3880,.T.);
#7111=EDGE_CURVE('',#5733,#5734,#3437,.T.);
#7112=EDGE_CURVE('',#5734,#5735,#3881,.T.);
#7113=EDGE_CURVE('',#5735,#5736,#3882,.T.);
#7114=EDGE_CURVE('',#5737,#5736,#3883,.T.);
#7115=EDGE_CURVE('',#5737,#5699,#3884,.T.);
#7116=EDGE_CURVE('',#5738,#5739,#3885,.T.);
#7117=EDGE_CURVE('',#5739,#5737,#3886,.T.);
#7118=EDGE_CURVE('',#5736,#5738,#3887,.T.);
#7119=EDGE_CURVE('',#5735,#5740,#3888,.T.);
#7120=EDGE_CURVE('',#5738,#5740,#3889,.T.);
#7121=EDGE_CURVE('',#5741,#5742,#3890,.T.);
#7122=EDGE_CURVE('',#5742,#5731,#3891,.T.);
#7123=EDGE_CURVE('',#5730,#5741,#3892,.T.);
#7124=EDGE_CURVE('',#5743,#5729,#3893,.T.);
#7125=EDGE_CURVE('',#5741,#5743,#3894,.T.);
#7126=EDGE_CURVE('',#5744,#5743,#3895,.T.);
#7127=EDGE_CURVE('',#5728,#5744,#3896,.T.);
#7128=EDGE_CURVE('',#5725,#5745,#3897,.T.);
#7129=EDGE_CURVE('',#5746,#5745,#3438,.T.);
#7130=EDGE_CURVE('',#5726,#5746,#3898,.T.);
#7131=EDGE_CURVE('',#5747,#5746,#3899,.T.);
#7132=EDGE_CURVE('',#5727,#5747,#3900,.T.);
#7133=EDGE_CURVE('',#5744,#5747,#3901,.T.);
#7134=EDGE_CURVE('',#5748,#5742,#3902,.T.);
#7135=EDGE_CURVE('',#5732,#5748,#3903,.T.);
#7136=EDGE_CURVE('',#5749,#5748,#3904,.T.);
#7137=EDGE_CURVE('',#5733,#5749,#3905,.T.);
#7138=EDGE_CURVE('',#5750,#5749,#3439,.T.);
#7139=EDGE_CURVE('',#5734,#5750,#3906,.T.);
#7140=EDGE_CURVE('',#5740,#5750,#3907,.T.);
#7141=EDGE_CURVE('',#5700,#5739,#3908,.T.);
#7142=EDGE_CURVE('',#5751,#5721,#3909,.T.);
#7143=EDGE_CURVE('',#5724,#5751,#3910,.T.);
#7144=EDGE_CURVE('',#5745,#5751,#3911,.T.);
#8965=ORIENTED_EDGE('',*,*,#7017,.F.);
#8966=ORIENTED_EDGE('',*,*,#7018,.T.);
#8967=ORIENTED_EDGE('',*,*,#7019,.T.);
#8968=ORIENTED_EDGE('',*,*,#7018,.F.);
#8969=ORIENTED_EDGE('',*,*,#7019,.F.);
#8970=ORIENTED_EDGE('',*,*,#7020,.T.);
#8971=ORIENTED_EDGE('',*,*,#7020,.F.);
#8972=ORIENTED_EDGE('',*,*,#7021,.T.);
#8973=ORIENTED_EDGE('',*,*,#7022,.F.);
#8974=ORIENTED_EDGE('',*,*,#7023,.F.);
#8975=ORIENTED_EDGE('',*,*,#7021,.F.);
#8976=ORIENTED_EDGE('',*,*,#7024,.F.);
#8977=ORIENTED_EDGE('',*,*,#7025,.T.);
#8978=ORIENTED_EDGE('',*,*,#7026,.T.);
#8979=ORIENTED_EDGE('',*,*,#7025,.F.);
#8980=ORIENTED_EDGE('',*,*,#7026,.F.);
#8981=ORIENTED_EDGE('',*,*,#7027,.T.);
#8982=ORIENTED_EDGE('',*,*,#7027,.F.);
#8983=ORIENTED_EDGE('',*,*,#7028,.T.);
#8984=ORIENTED_EDGE('',*,*,#7029,.F.);
#8985=ORIENTED_EDGE('',*,*,#7030,.F.);
#8986=ORIENTED_EDGE('',*,*,#7028,.F.);
#8987=ORIENTED_EDGE('',*,*,#7031,.F.);
#8988=ORIENTED_EDGE('',*,*,#7032,.T.);
#8989=ORIENTED_EDGE('',*,*,#7033,.T.);
#8990=ORIENTED_EDGE('',*,*,#7032,.F.);
#8991=ORIENTED_EDGE('',*,*,#7033,.F.);
#8992=ORIENTED_EDGE('',*,*,#7034,.T.);
#8993=ORIENTED_EDGE('',*,*,#7034,.F.);
#8994=ORIENTED_EDGE('',*,*,#7035,.T.);
#8995=ORIENTED_EDGE('',*,*,#7036,.F.);
#8996=ORIENTED_EDGE('',*,*,#7037,.F.);
#8997=ORIENTED_EDGE('',*,*,#7035,.F.);
#8998=ORIENTED_EDGE('',*,*,#7038,.F.);
#8999=ORIENTED_EDGE('',*,*,#7039,.T.);
#9000=ORIENTED_EDGE('',*,*,#7040,.T.);
#9001=ORIENTED_EDGE('',*,*,#7039,.F.);
#9002=ORIENTED_EDGE('',*,*,#7040,.F.);
#9003=ORIENTED_EDGE('',*,*,#7041,.T.);
#9004=ORIENTED_EDGE('',*,*,#7041,.F.);
#9005=ORIENTED_EDGE('',*,*,#7042,.T.);
#9006=ORIENTED_EDGE('',*,*,#7043,.F.);
#9007=ORIENTED_EDGE('',*,*,#7044,.F.);
#9008=ORIENTED_EDGE('',*,*,#7042,.F.);
#9009=ORIENTED_EDGE('',*,*,#7045,.F.);
#9010=ORIENTED_EDGE('',*,*,#7046,.T.);
#9011=ORIENTED_EDGE('',*,*,#7047,.T.);
#9012=ORIENTED_EDGE('',*,*,#7046,.F.);
#9013=ORIENTED_EDGE('',*,*,#7047,.F.);
#9014=ORIENTED_EDGE('',*,*,#7048,.T.);
#9015=ORIENTED_EDGE('',*,*,#7048,.F.);
#9016=ORIENTED_EDGE('',*,*,#7049,.T.);
#9017=ORIENTED_EDGE('',*,*,#7050,.F.);
#9018=ORIENTED_EDGE('',*,*,#7051,.F.);
#9019=ORIENTED_EDGE('',*,*,#7049,.F.);
#9020=ORIENTED_EDGE('',*,*,#7052,.F.);
#9021=ORIENTED_EDGE('',*,*,#7053,.T.);
#9022=ORIENTED_EDGE('',*,*,#7054,.T.);
#9023=ORIENTED_EDGE('',*,*,#7053,.F.);
#9024=ORIENTED_EDGE('',*,*,#7054,.F.);
#9025=ORIENTED_EDGE('',*,*,#7055,.T.);
#9026=ORIENTED_EDGE('',*,*,#7055,.F.);
#9027=ORIENTED_EDGE('',*,*,#7056,.T.);
#9028=ORIENTED_EDGE('',*,*,#7057,.F.);
#9029=ORIENTED_EDGE('',*,*,#7058,.F.);
#9030=ORIENTED_EDGE('',*,*,#7056,.F.);
#9031=ORIENTED_EDGE('',*,*,#7059,.T.);
#9032=ORIENTED_EDGE('',*,*,#7060,.T.);
#9033=ORIENTED_EDGE('',*,*,#7061,.T.);
#9034=ORIENTED_EDGE('',*,*,#7060,.F.);
#9035=ORIENTED_EDGE('',*,*,#7062,.T.);
#9036=ORIENTED_EDGE('',*,*,#7063,.T.);
#9037=ORIENTED_EDGE('',*,*,#7064,.F.);
#9038=ORIENTED_EDGE('',*,*,#7065,.F.);
#9039=ORIENTED_EDGE('',*,*,#7066,.F.);
#9040=ORIENTED_EDGE('',*,*,#7067,.F.);
#9041=ORIENTED_EDGE('',*,*,#7068,.F.);
#9042=ORIENTED_EDGE('',*,*,#7061,.F.);
#9043=ORIENTED_EDGE('',*,*,#7059,.F.);
#9044=ORIENTED_EDGE('',*,*,#7069,.T.);
#9045=ORIENTED_EDGE('',*,*,#7070,.T.);
#9046=ORIENTED_EDGE('',*,*,#7069,.F.);
#9047=ORIENTED_EDGE('',*,*,#7071,.T.);
#9048=ORIENTED_EDGE('',*,*,#7072,.T.);
#9049=ORIENTED_EDGE('',*,*,#7066,.T.);
#9050=ORIENTED_EDGE('',*,*,#7072,.F.);
#9051=ORIENTED_EDGE('',*,*,#7071,.F.);
#9052=ORIENTED_EDGE('',*,*,#7073,.T.);
#9053=ORIENTED_EDGE('',*,*,#7074,.T.);
#9054=ORIENTED_EDGE('',*,*,#7073,.F.);
#9055=ORIENTED_EDGE('',*,*,#7075,.T.);
#9056=ORIENTED_EDGE('',*,*,#7076,.T.);
#9057=ORIENTED_EDGE('',*,*,#7068,.T.);
#9058=ORIENTED_EDGE('',*,*,#7076,.F.);
#9059=ORIENTED_EDGE('',*,*,#7075,.F.);
#9060=ORIENTED_EDGE('',*,*,#7077,.T.);
#9061=ORIENTED_EDGE('',*,*,#7078,.T.);
#9062=ORIENTED_EDGE('',*,*,#7077,.F.);
#9063=ORIENTED_EDGE('',*,*,#7079,.T.);
#9064=ORIENTED_EDGE('',*,*,#7080,.T.);
#9065=ORIENTED_EDGE('',*,*,#7067,.T.);
#9066=ORIENTED_EDGE('',*,*,#7080,.F.);
#9067=ORIENTED_EDGE('',*,*,#7079,.F.);
#9068=ORIENTED_EDGE('',*,*,#7081,.T.);
#9069=ORIENTED_EDGE('',*,*,#7082,.T.);
#9070=ORIENTED_EDGE('',*,*,#7081,.F.);
#9071=ORIENTED_EDGE('',*,*,#7082,.F.);
#9072=ORIENTED_EDGE('',*,*,#7083,.F.);
#9073=ORIENTED_EDGE('',*,*,#7078,.F.);
#9074=ORIENTED_EDGE('',*,*,#7084,.F.);
#9075=ORIENTED_EDGE('',*,*,#7074,.F.);
#9076=ORIENTED_EDGE('',*,*,#7085,.F.);
#9077=ORIENTED_EDGE('',*,*,#7070,.F.);
#9078=ORIENTED_EDGE('',*,*,#7086,.F.);
#9079=ORIENTED_EDGE('',*,*,#7083,.T.);
#9080=ORIENTED_EDGE('',*,*,#7087,.T.);
#9081=ORIENTED_EDGE('',*,*,#7088,.F.);
#9082=ORIENTED_EDGE('',*,*,#7087,.F.);
#9083=ORIENTED_EDGE('',*,*,#7084,.T.);
#9084=ORIENTED_EDGE('',*,*,#7089,.T.);
#9085=ORIENTED_EDGE('',*,*,#7090,.F.);
#9086=ORIENTED_EDGE('',*,*,#7089,.F.);
#9087=ORIENTED_EDGE('',*,*,#7085,.T.);
#9088=ORIENTED_EDGE('',*,*,#7091,.T.);
#9089=ORIENTED_EDGE('',*,*,#7092,.F.);
#9090=ORIENTED_EDGE('',*,*,#7091,.F.);
#9091=ORIENTED_EDGE('',*,*,#7086,.T.);
#9092=ORIENTED_EDGE('',*,*,#7093,.T.);
#9093=ORIENTED_EDGE('',*,*,#7094,.F.);
#9094=ORIENTED_EDGE('',*,*,#7093,.F.);
#9095=ORIENTED_EDGE('',*,*,#7095,.T.);
#9096=ORIENTED_EDGE('',*,*,#7096,.T.);
#9097=ORIENTED_EDGE('',*,*,#7097,.T.);
#9098=ORIENTED_EDGE('',*,*,#7098,.T.);
#9099=ORIENTED_EDGE('',*,*,#7098,.F.);
#9100=ORIENTED_EDGE('',*,*,#7099,.T.);
#9101=ORIENTED_EDGE('',*,*,#7065,.T.);
#9102=ORIENTED_EDGE('',*,*,#7100,.F.);
#9103=ORIENTED_EDGE('',*,*,#7097,.F.);
#9104=ORIENTED_EDGE('',*,*,#7101,.F.);
#9105=ORIENTED_EDGE('',*,*,#7102,.F.);
#9106=ORIENTED_EDGE('',*,*,#7103,.T.);
#9107=ORIENTED_EDGE('',*,*,#7104,.F.);
#9108=ORIENTED_EDGE('',*,*,#7105,.F.);
#9109=ORIENTED_EDGE('',*,*,#7106,.F.);
#9110=ORIENTED_EDGE('',*,*,#7107,.T.);
#9111=ORIENTED_EDGE('',*,*,#7108,.F.);
#9112=ORIENTED_EDGE('',*,*,#7109,.T.);
#9113=ORIENTED_EDGE('',*,*,#7110,.T.);
#9114=ORIENTED_EDGE('',*,*,#7111,.T.);
#9115=ORIENTED_EDGE('',*,*,#7112,.T.);
#9116=ORIENTED_EDGE('',*,*,#7113,.T.);
#9117=ORIENTED_EDGE('',*,*,#7114,.F.);
#9118=ORIENTED_EDGE('',*,*,#7115,.T.);
#9119=ORIENTED_EDGE('',*,*,#7062,.F.);
#9120=ORIENTED_EDGE('',*,*,#7099,.F.);
#9121=ORIENTED_EDGE('',*,*,#7116,.T.);
#9122=ORIENTED_EDGE('',*,*,#7117,.T.);
#9123=ORIENTED_EDGE('',*,*,#7114,.T.);
#9124=ORIENTED_EDGE('',*,*,#7118,.T.);
#9125=ORIENTED_EDGE('',*,*,#7118,.F.);
#9126=ORIENTED_EDGE('',*,*,#7113,.F.);
#9127=ORIENTED_EDGE('',*,*,#7119,.T.);
#9128=ORIENTED_EDGE('',*,*,#7120,.F.);
#9129=ORIENTED_EDGE('',*,*,#7121,.T.);
#9130=ORIENTED_EDGE('',*,*,#7122,.T.);
#9131=ORIENTED_EDGE('',*,*,#7108,.T.);
#9132=ORIENTED_EDGE('',*,*,#7123,.T.);
#9133=ORIENTED_EDGE('',*,*,#7123,.F.);
#9134=ORIENTED_EDGE('',*,*,#7107,.F.);
#9135=ORIENTED_EDGE('',*,*,#7124,.F.);
#9136=ORIENTED_EDGE('',*,*,#7125,.F.);
#9137=ORIENTED_EDGE('',*,*,#7024,.T.);
#9138=ORIENTED_EDGE('',*,*,#7094,.T.);
#9139=ORIENTED_EDGE('',*,*,#7092,.T.);
#9140=ORIENTED_EDGE('',*,*,#7090,.T.);
#9141=ORIENTED_EDGE('',*,*,#7088,.T.);
#9142=ORIENTED_EDGE('',*,*,#7052,.T.);
#9143=ORIENTED_EDGE('',*,*,#7045,.T.);
#9144=ORIENTED_EDGE('',*,*,#7038,.T.);
#9145=ORIENTED_EDGE('',*,*,#7031,.T.);
#9146=ORIENTED_EDGE('',*,*,#7017,.T.);
#9147=ORIENTED_EDGE('',*,*,#7126,.T.);
#9148=ORIENTED_EDGE('',*,*,#7124,.T.);
#9149=ORIENTED_EDGE('',*,*,#7106,.T.);
#9150=ORIENTED_EDGE('',*,*,#7127,.T.);
#9151=ORIENTED_EDGE('',*,*,#7103,.F.);
#9152=ORIENTED_EDGE('',*,*,#7128,.T.);
#9153=ORIENTED_EDGE('',*,*,#7129,.F.);
#9154=ORIENTED_EDGE('',*,*,#7130,.F.);
#9155=ORIENTED_EDGE('',*,*,#7022,.T.);
#9156=ORIENTED_EDGE('',*,*,#7023,.T.);
#9157=ORIENTED_EDGE('',*,*,#7029,.T.);
#9158=ORIENTED_EDGE('',*,*,#7030,.T.);
#9159=ORIENTED_EDGE('',*,*,#7036,.T.);
#9160=ORIENTED_EDGE('',*,*,#7037,.T.);
#9161=ORIENTED_EDGE('',*,*,#7104,.T.);
#9162=ORIENTED_EDGE('',*,*,#7130,.T.);
#9163=ORIENTED_EDGE('',*,*,#7131,.F.);
#9164=ORIENTED_EDGE('',*,*,#7132,.F.);
#9165=ORIENTED_EDGE('',*,*,#7127,.F.);
#9166=ORIENTED_EDGE('',*,*,#7105,.T.);
#9167=ORIENTED_EDGE('',*,*,#7132,.T.);
#9168=ORIENTED_EDGE('',*,*,#7133,.F.);
#9169=ORIENTED_EDGE('',*,*,#7122,.F.);
#9170=ORIENTED_EDGE('',*,*,#7134,.F.);
#9171=ORIENTED_EDGE('',*,*,#7135,.F.);
#9172=ORIENTED_EDGE('',*,*,#7109,.F.);
#9173=ORIENTED_EDGE('',*,*,#7110,.F.);
#9174=ORIENTED_EDGE('',*,*,#7135,.T.);
#9175=ORIENTED_EDGE('',*,*,#7136,.F.);
#9176=ORIENTED_EDGE('',*,*,#7137,.F.);
#9177=ORIENTED_EDGE('',*,*,#7111,.F.);
#9178=ORIENTED_EDGE('',*,*,#7137,.T.);
#9179=ORIENTED_EDGE('',*,*,#7138,.F.);
#9180=ORIENTED_EDGE('',*,*,#7139,.F.);
#9181=ORIENTED_EDGE('',*,*,#7043,.T.);
#9182=ORIENTED_EDGE('',*,*,#7044,.T.);
#9183=ORIENTED_EDGE('',*,*,#7050,.T.);
#9184=ORIENTED_EDGE('',*,*,#7051,.T.);
#9185=ORIENTED_EDGE('',*,*,#7057,.T.);
#9186=ORIENTED_EDGE('',*,*,#7058,.T.);
#9187=ORIENTED_EDGE('',*,*,#7112,.F.);
#9188=ORIENTED_EDGE('',*,*,#7139,.T.);
#9189=ORIENTED_EDGE('',*,*,#7140,.F.);
#9190=ORIENTED_EDGE('',*,*,#7119,.F.);
#9191=ORIENTED_EDGE('',*,*,#7117,.F.);
#9192=ORIENTED_EDGE('',*,*,#7141,.F.);
#9193=ORIENTED_EDGE('',*,*,#7063,.F.);
#9194=ORIENTED_EDGE('',*,*,#7115,.F.);
#9195=ORIENTED_EDGE('',*,*,#7096,.F.);
#9196=ORIENTED_EDGE('',*,*,#7142,.F.);
#9197=ORIENTED_EDGE('',*,*,#7143,.F.);
#9198=ORIENTED_EDGE('',*,*,#7101,.T.);
#9199=ORIENTED_EDGE('',*,*,#7102,.T.);
#9200=ORIENTED_EDGE('',*,*,#7143,.T.);
#9201=ORIENTED_EDGE('',*,*,#7144,.F.);
#9202=ORIENTED_EDGE('',*,*,#7128,.F.);
#9203=ORIENTED_EDGE('',*,*,#7095,.F.);
#9204=ORIENTED_EDGE('',*,*,#7100,.T.);
#9205=ORIENTED_EDGE('',*,*,#7064,.T.);
#9206=ORIENTED_EDGE('',*,*,#7141,.T.);
#9207=ORIENTED_EDGE('',*,*,#7116,.F.);
#9208=ORIENTED_EDGE('',*,*,#7120,.T.);
#9209=ORIENTED_EDGE('',*,*,#7140,.T.);
#9210=ORIENTED_EDGE('',*,*,#7138,.T.);
#9211=ORIENTED_EDGE('',*,*,#7136,.T.);
#9212=ORIENTED_EDGE('',*,*,#7134,.T.);
#9213=ORIENTED_EDGE('',*,*,#7121,.F.);
#9214=ORIENTED_EDGE('',*,*,#7125,.T.);
#9215=ORIENTED_EDGE('',*,*,#7126,.F.);
#9216=ORIENTED_EDGE('',*,*,#7133,.T.);
#9217=ORIENTED_EDGE('',*,*,#7131,.T.);
#9218=ORIENTED_EDGE('',*,*,#7129,.T.);
#9219=ORIENTED_EDGE('',*,*,#7144,.T.);
#9220=ORIENTED_EDGE('',*,*,#7142,.T.);
#12861=CYLINDRICAL_SURFACE('',#13758,4.25);
#12862=CYLINDRICAL_SURFACE('',#13763,2.6);
#12863=CYLINDRICAL_SURFACE('',#13764,4.25);
#12864=CYLINDRICAL_SURFACE('',#13769,2.6);
#12865=CYLINDRICAL_SURFACE('',#13770,4.25);
#12866=CYLINDRICAL_SURFACE('',#13775,2.6);
#12867=CYLINDRICAL_SURFACE('',#13776,4.25);
#12868=CYLINDRICAL_SURFACE('',#13781,2.6);
#12869=CYLINDRICAL_SURFACE('',#13782,4.25);
#12870=CYLINDRICAL_SURFACE('',#13787,2.6);
#12871=CYLINDRICAL_SURFACE('',#13788,4.25);
#12872=CYLINDRICAL_SURFACE('',#13793,2.6);
#12873=CYLINDRICAL_SURFACE('',#13801,5.35);
#12874=CYLINDRICAL_SURFACE('',#13805,5.35);
#12875=CYLINDRICAL_SURFACE('',#13809,5.35);
#12876=CYLINDRICAL_SURFACE('',#13813,5.35);
#12877=CYLINDRICAL_SURFACE('',#13823,3.55600000000001);
#12878=CYLINDRICAL_SURFACE('',#13825,3.556);
#12879=CYLINDRICAL_SURFACE('',#13827,3.556);
#12880=CYLINDRICAL_SURFACE('',#13829,3.55600000000001);
#12881=CYLINDRICAL_SURFACE('',#13841,6.35);
#12882=CYLINDRICAL_SURFACE('',#13847,6.35);
#12987=ADVANCED_FACE('',(#2027),#12861,.F.);
#12988=ADVANCED_FACE('',(#2028,#1484),#1565,.F.);
#12989=ADVANCED_FACE('',(#2029),#12862,.F.);
#12990=ADVANCED_FACE('',(#2030),#12863,.F.);
#12991=ADVANCED_FACE('',(#2031,#1485),#1566,.F.);
#12992=ADVANCED_FACE('',(#2032),#12864,.F.);
#12993=ADVANCED_FACE('',(#2033),#12865,.F.);
#12994=ADVANCED_FACE('',(#2034,#1486),#1567,.F.);
#12995=ADVANCED_FACE('',(#2035),#12866,.F.);
#12996=ADVANCED_FACE('',(#2036),#12867,.F.);
#12997=ADVANCED_FACE('',(#2037,#1487),#1568,.F.);
#12998=ADVANCED_FACE('',(#2038),#12868,.F.);
#12999=ADVANCED_FACE('',(#2039),#12869,.F.);
#13000=ADVANCED_FACE('',(#2040,#1488),#1569,.F.);
#13001=ADVANCED_FACE('',(#2041),#12870,.F.);
#13002=ADVANCED_FACE('',(#2042),#12871,.F.);
#13003=ADVANCED_FACE('',(#2043,#1489),#1570,.F.);
#13004=ADVANCED_FACE('',(#2044),#12872,.F.);
#13005=ADVANCED_FACE('',(#2045),#1053,.F.);
#13006=ADVANCED_FACE('',(#2046,#1490,#1491,#1492,#1493),#1571,.T.);
#13007=ADVANCED_FACE('',(#2047),#12873,.F.);
#13008=ADVANCED_FACE('',(#2048),#1054,.F.);
#13009=ADVANCED_FACE('',(#2049),#12874,.F.);
#13010=ADVANCED_FACE('',(#2050),#1055,.F.);
#13011=ADVANCED_FACE('',(#2051),#12875,.F.);
#13012=ADVANCED_FACE('',(#2052),#1056,.F.);
#13013=ADVANCED_FACE('',(#2053),#12876,.F.);
#13014=ADVANCED_FACE('',(#2054,#1494),#1572,.T.);
#13015=ADVANCED_FACE('',(#2055,#1495),#1573,.T.);
#13016=ADVANCED_FACE('',(#2056,#1496),#1574,.T.);
#13017=ADVANCED_FACE('',(#2057,#1497),#1575,.T.);
#13018=ADVANCED_FACE('',(#2058),#12877,.F.);
#13019=ADVANCED_FACE('',(#2059),#12878,.F.);
#13020=ADVANCED_FACE('',(#2060),#12879,.F.);
#13021=ADVANCED_FACE('',(#2061),#12880,.F.);
#13022=ADVANCED_FACE('',(#2062),#1576,.T.);
#13023=ADVANCED_FACE('',(#2063),#1577,.T.);
#13024=ADVANCED_FACE('',(#2064),#1578,.F.);
#13025=ADVANCED_FACE('',(#2065),#1579,.T.);
#13026=ADVANCED_FACE('',(#2066),#1580,.T.);
#13027=ADVANCED_FACE('',(#2067),#1581,.T.);
#13028=ADVANCED_FACE('',(#2068,#1498,#1499,#1500,#1501,#1502,#1503,#1504,
#1505,#1506,#1507),#1582,.T.);
#13029=ADVANCED_FACE('',(#2069),#1583,.T.);
#13030=ADVANCED_FACE('',(#2070,#1508,#1509,#1510),#12881,.F.);
#13031=ADVANCED_FACE('',(#2071),#1584,.T.);
#13032=ADVANCED_FACE('',(#2072),#1585,.T.);
#13033=ADVANCED_FACE('',(#2073),#1586,.T.);
#13034=ADVANCED_FACE('',(#2074),#1587,.T.);
#13035=ADVANCED_FACE('',(#2075,#1511,#1512,#1513),#12882,.F.);
#13036=ADVANCED_FACE('',(#2076),#1588,.T.);
#13037=ADVANCED_FACE('',(#2077),#1589,.T.);
#13038=ADVANCED_FACE('',(#2078),#1590,.T.);
#13039=ADVANCED_FACE('',(#2079),#1591,.T.);
#13040=ADVANCED_FACE('',(#2080),#1592,.T.);
#13635=CLOSED_SHELL('',(#12987,#12988,#12989,#12990,#12991,#12992,#12993,
#12994,#12995,#12996,#12997,#12998,#12999,#13000,#13001,#13002,#13003,#13004,
#13005,#13006,#13007,#13008,#13009,#13010,#13011,#13012,#13013,#13014,#13015,
#13016,#13017,#13018,#13019,#13020,#13021,#13022,#13023,#13024,#13025,#13026,
#13027,#13028,#13029,#13030,#13031,#13032,#13033,#13034,#13035,#13036,#13037,
#13038,#13039,#13040));
#13757=AXIS2_PLACEMENT_3D('',#18529,#15045,#15046);
#13758=AXIS2_PLACEMENT_3D('',#18530,#15047,#15048);
#13759=AXIS2_PLACEMENT_3D('',#18532,#15049,#15050);
#13760=AXIS2_PLACEMENT_3D('',#18535,#15052,#15053);
#13761=AXIS2_PLACEMENT_3D('',#18536,#15054,#15055);
#13762=AXIS2_PLACEMENT_3D('',#18538,#15056,#15057);
#13763=AXIS2_PLACEMENT_3D('',#18539,#15058,#15059);
#13764=AXIS2_PLACEMENT_3D('',#18579,#15061,#15062);
#13765=AXIS2_PLACEMENT_3D('',#18581,#15063,#15064);
#13766=AXIS2_PLACEMENT_3D('',#18584,#15066,#15067);
#13767=AXIS2_PLACEMENT_3D('',#18585,#15068,#15069);
#13768=AXIS2_PLACEMENT_3D('',#18587,#15070,#15071);
#13769=AXIS2_PLACEMENT_3D('',#18588,#15072,#15073);
#13770=AXIS2_PLACEMENT_3D('',#18628,#15075,#15076);
#13771=AXIS2_PLACEMENT_3D('',#18630,#15077,#15078);
#13772=AXIS2_PLACEMENT_3D('',#18633,#15080,#15081);
#13773=AXIS2_PLACEMENT_3D('',#18634,#15082,#15083);
#13774=AXIS2_PLACEMENT_3D('',#18636,#15084,#15085);
#13775=AXIS2_PLACEMENT_3D('',#18637,#15086,#15087);
#13776=AXIS2_PLACEMENT_3D('',#18677,#15089,#15090);
#13777=AXIS2_PLACEMENT_3D('',#18679,#15091,#15092);
#13778=AXIS2_PLACEMENT_3D('',#18682,#15094,#15095);
#13779=AXIS2_PLACEMENT_3D('',#18683,#15096,#15097);
#13780=AXIS2_PLACEMENT_3D('',#18685,#15098,#15099);
#13781=AXIS2_PLACEMENT_3D('',#18686,#15100,#15101);
#13782=AXIS2_PLACEMENT_3D('',#18726,#15103,#15104);
#13783=AXIS2_PLACEMENT_3D('',#18728,#15105,#15106);
#13784=AXIS2_PLACEMENT_3D('',#18731,#15108,#15109);
#13785=AXIS2_PLACEMENT_3D('',#18732,#15110,#15111);
#13786=AXIS2_PLACEMENT_3D('',#18734,#15112,#15113);
#13787=AXIS2_PLACEMENT_3D('',#18735,#15114,#15115);
#13788=AXIS2_PLACEMENT_3D('',#18775,#15117,#15118);
#13789=AXIS2_PLACEMENT_3D('',#18777,#15119,#15120);
#13790=AXIS2_PLACEMENT_3D('',#18780,#15122,#15123);
#13791=AXIS2_PLACEMENT_3D('',#18781,#15124,#15125);
#13792=AXIS2_PLACEMENT_3D('',#18783,#15126,#15127);
#13793=AXIS2_PLACEMENT_3D('',#18784,#15128,#15129);
#13794=AXIS2_PLACEMENT_3D('',#18824,#15131,#15132);
#13795=AXIS2_PLACEMENT_3D('',#18826,#15133,#15134);
#13796=AXIS2_PLACEMENT_3D('',#18829,#15136,#15137);
#13797=AXIS2_PLACEMENT_3D('',#18830,#15138,#15139);
#13798=AXIS2_PLACEMENT_3D('',#18840,#15144,#15145);
#13799=AXIS2_PLACEMENT_3D('',#18842,#15146,#15147);
#13800=AXIS2_PLACEMENT_3D('',#18844,#15148,#15149);
#13801=AXIS2_PLACEMENT_3D('',#18845,#15150,#15151);
#13802=AXIS2_PLACEMENT_3D('',#18848,#15153,#15154);
#13803=AXIS2_PLACEMENT_3D('',#18849,#15155,#15156);
#13804=AXIS2_PLACEMENT_3D('',#18851,#15157,#15158);
#13805=AXIS2_PLACEMENT_3D('',#18853,#15160,#15161);
#13806=AXIS2_PLACEMENT_3D('',#18856,#15163,#15164);
#13807=AXIS2_PLACEMENT_3D('',#18857,#15165,#15166);
#13808=AXIS2_PLACEMENT_3D('',#18859,#15167,#15168);
#13809=AXIS2_PLACEMENT_3D('',#18861,#15170,#15171);
#13810=AXIS2_PLACEMENT_3D('',#18864,#15173,#15174);
#13811=AXIS2_PLACEMENT_3D('',#18865,#15175,#15176);
#13812=AXIS2_PLACEMENT_3D('',#18867,#15177,#15178);
#13813=AXIS2_PLACEMENT_3D('',#18869,#15180,#15181);
#13814=AXIS2_PLACEMENT_3D('',#18872,#15183,#15184);
#13815=AXIS2_PLACEMENT_3D('',#18873,#15185,#15186);
#13816=AXIS2_PLACEMENT_3D('',#18875,#15187,#15188);
#13817=AXIS2_PLACEMENT_3D('',#18876,#15189,#15190);
#13818=AXIS2_PLACEMENT_3D('',#18878,#15191,#15192);
#13819=AXIS2_PLACEMENT_3D('',#18879,#15193,#15194);
#13820=AXIS2_PLACEMENT_3D('',#18881,#15195,#15196);
#13821=AXIS2_PLACEMENT_3D('',#18882,#15197,#15198);
#13822=AXIS2_PLACEMENT_3D('',#18884,#15199,#15200);
#13823=AXIS2_PLACEMENT_3D('',#18885,#15201,#15202);
#13824=AXIS2_PLACEMENT_3D('',#18888,#15204,#15205);
#13825=AXIS2_PLACEMENT_3D('',#18889,#15206,#15207);
#13826=AXIS2_PLACEMENT_3D('',#18892,#15209,#15210);
#13827=AXIS2_PLACEMENT_3D('',#18893,#15211,#15212);
#13828=AXIS2_PLACEMENT_3D('',#18896,#15214,#15215);
#13829=AXIS2_PLACEMENT_3D('',#18897,#15216,#15217);
#13830=AXIS2_PLACEMENT_3D('',#18900,#15219,#15220);
#13831=AXIS2_PLACEMENT_3D('',#18901,#15221,#15222);
#13832=AXIS2_PLACEMENT_3D('',#18910,#15227,#15228);
#13833=AXIS2_PLACEMENT_3D('',#18913,#15231,#15232);
#13834=AXIS2_PLACEMENT_3D('',#18919,#15235,#15236);
#13835=AXIS2_PLACEMENT_3D('',#18935,#15244,#15245);
#13836=AXIS2_PLACEMENT_3D('',#18943,#15250,#15251);
#13837=AXIS2_PLACEMENT_3D('',#18949,#15255,#15256);
#13838=AXIS2_PLACEMENT_3D('',#18953,#15259,#15260);
#13839=AXIS2_PLACEMENT_3D('',#18959,#15264,#15265);
#13840=AXIS2_PLACEMENT_3D('',#18963,#15268,#15269);
#13841=AXIS2_PLACEMENT_3D('',#18967,#15272,#15273);
#13842=AXIS2_PLACEMENT_3D('',#18971,#15275,#15276);
#13843=AXIS2_PLACEMENT_3D('',#18973,#15278,#15279);
#13844=AXIS2_PLACEMENT_3D('',#18977,#15282,#15283);
#13845=AXIS2_PLACEMENT_3D('',#18979,#15285,#15286);
#13846=AXIS2_PLACEMENT_3D('',#18983,#15289,#15290);
#13847=AXIS2_PLACEMENT_3D('',#18987,#15293,#15294);
#13848=AXIS2_PLACEMENT_3D('',#18989,#15295,#15296);
#13849=AXIS2_PLACEMENT_3D('',#18991,#15298,#15299);
#13850=AXIS2_PLACEMENT_3D('',#18993,#15301,#15302);
#13851=AXIS2_PLACEMENT_3D('',#18995,#15304,#15305);
#13852=AXIS2_PLACEMENT_3D('',#18999,#15308,#15309);
#13853=AXIS2_PLACEMENT_3D('',#19001,#15311,#15312);
#15045=DIRECTION('axis',(0.,0.,1.));
#15046=DIRECTION('refdir',(1.,0.,0.));
#15047=DIRECTION('center_axis',(0.,0.707106781186547,-0.707106781186548));
#15048=DIRECTION('ref_axis',(0.,0.707106781186548,0.707106781186547));
#15049=DIRECTION('center_axis',(0.,1.,0.));
#15050=DIRECTION('ref_axis',(0.,0.,1.));
#15051=DIRECTION('',(0.,0.707106781186547,-0.707106781186548));
#15052=DIRECTION('center_axis',(0.,0.707106781186547,-0.707106781186548));
#15053=DIRECTION('ref_axis',(1.,0.,0.));
#15054=DIRECTION('center_axis',(0.,0.707106781186547,-0.707106781186548));
#15055=DIRECTION('ref_axis',(-1.,0.,0.));
#15056=DIRECTION('center_axis',(0.,0.707106781186547,-0.707106781186548));
#15057=DIRECTION('ref_axis',(1.,0.,0.));
#15058=DIRECTION('center_axis',(0.,0.707106781186547,-0.707106781186548));
#15059=DIRECTION('ref_axis',(0.,0.707106781186548,0.707106781186547));
#15060=DIRECTION('',(0.,0.707106781186547,-0.707106781186548));
#15061=DIRECTION('center_axis',(0.,0.707106781186547,-0.707106781186548));
#15062=DIRECTION('ref_axis',(0.,0.707106781186548,0.707106781186547));
#15063=DIRECTION('center_axis',(0.,1.,0.));
#15064=DIRECTION('ref_axis',(0.,0.,1.));
#15065=DIRECTION('',(0.,0.707106781186547,-0.707106781186548));
#15066=DIRECTION('center_axis',(0.,0.707106781186547,-0.707106781186548));
#15067=DIRECTION('ref_axis',(1.,0.,0.));
#15068=DIRECTION('center_axis',(0.,0.707106781186547,-0.707106781186548));
#15069=DIRECTION('ref_axis',(-1.,0.,0.));
#15070=DIRECTION('center_axis',(0.,0.707106781186547,-0.707106781186548));
#15071=DIRECTION('ref_axis',(1.,0.,0.));
#15072=DIRECTION('center_axis',(0.,0.707106781186547,-0.707106781186548));
#15073=DIRECTION('ref_axis',(0.,0.707106781186548,0.707106781186547));
#15074=DIRECTION('',(0.,0.707106781186547,-0.707106781186548));
#15075=DIRECTION('center_axis',(0.,0.707106781186547,-0.707106781186548));
#15076=DIRECTION('ref_axis',(0.,0.707106781186548,0.707106781186547));
#15077=DIRECTION('center_axis',(0.,1.,0.));
#15078=DIRECTION('ref_axis',(0.,0.,1.));
#15079=DIRECTION('',(0.,0.707106781186547,-0.707106781186548));
#15080=DIRECTION('center_axis',(0.,0.707106781186547,-0.707106781186548));
#15081=DIRECTION('ref_axis',(1.,0.,0.));
#15082=DIRECTION('center_axis',(0.,0.707106781186547,-0.707106781186548));
#15083=DIRECTION('ref_axis',(-1.,0.,0.));
#15084=DIRECTION('center_axis',(0.,0.707106781186547,-0.707106781186548));
#15085=DIRECTION('ref_axis',(1.,0.,0.));
#15086=DIRECTION('center_axis',(0.,0.707106781186547,-0.707106781186548));
#15087=DIRECTION('ref_axis',(0.,0.707106781186548,0.707106781186547));
#15088=DIRECTION('',(0.,0.707106781186547,-0.707106781186548));
#15089=DIRECTION('center_axis',(0.,0.707106781186547,0.707106781186548));
#15090=DIRECTION('ref_axis',(0.,-0.707106781186548,0.707106781186547));
#15091=DIRECTION('center_axis',(0.,1.,0.));
#15092=DIRECTION('ref_axis',(0.,0.,1.));
#15093=DIRECTION('',(0.,0.707106781186547,0.707106781186548));
#15094=DIRECTION('center_axis',(0.,0.707106781186547,0.707106781186548));
#15095=DIRECTION('ref_axis',(1.,0.,0.));
#15096=DIRECTION('center_axis',(0.,0.707106781186547,0.707106781186548));
#15097=DIRECTION('ref_axis',(1.,0.,0.));
#15098=DIRECTION('center_axis',(0.,0.707106781186547,0.707106781186548));
#15099=DIRECTION('ref_axis',(1.,0.,0.));
#15100=DIRECTION('center_axis',(0.,0.707106781186547,0.707106781186548));
#15101=DIRECTION('ref_axis',(0.,-0.707106781186548,0.707106781186547));
#15102=DIRECTION('',(0.,0.707106781186547,0.707106781186548));
#15103=DIRECTION('center_axis',(0.,0.707106781186547,0.707106781186548));
#15104=DIRECTION('ref_axis',(0.,-0.707106781186548,0.707106781186547));
#15105=DIRECTION('center_axis',(0.,1.,0.));
#15106=DIRECTION('ref_axis',(0.,0.,1.));
#15107=DIRECTION('',(0.,0.707106781186547,0.707106781186548));
#15108=DIRECTION('center_axis',(0.,0.707106781186547,0.707106781186548));
#15109=DIRECTION('ref_axis',(1.,0.,0.));
#15110=DIRECTION('center_axis',(0.,0.707106781186547,0.707106781186548));
#15111=DIRECTION('ref_axis',(1.,0.,0.));
#15112=DIRECTION('center_axis',(0.,0.707106781186547,0.707106781186548));
#15113=DIRECTION('ref_axis',(1.,0.,0.));
#15114=DIRECTION('center_axis',(0.,0.707106781186547,0.707106781186548));
#15115=DIRECTION('ref_axis',(0.,-0.707106781186548,0.707106781186547));
#15116=DIRECTION('',(0.,0.707106781186547,0.707106781186548));
#15117=DIRECTION('center_axis',(0.,0.707106781186547,0.707106781186548));
#15118=DIRECTION('ref_axis',(0.,-0.707106781186548,0.707106781186547));
#15119=DIRECTION('center_axis',(0.,1.,0.));
#15120=DIRECTION('ref_axis',(0.,0.,1.));
#15121=DIRECTION('',(0.,0.707106781186547,0.707106781186548));
#15122=DIRECTION('center_axis',(0.,0.707106781186547,0.707106781186548));
#15123=DIRECTION('ref_axis',(1.,0.,0.));
#15124=DIRECTION('center_axis',(0.,0.707106781186547,0.707106781186548));
#15125=DIRECTION('ref_axis',(1.,0.,0.));
#15126=DIRECTION('center_axis',(0.,0.707106781186547,0.707106781186548));
#15127=DIRECTION('ref_axis',(1.,0.,0.));
#15128=DIRECTION('center_axis',(0.,0.707106781186547,0.707106781186548));
#15129=DIRECTION('ref_axis',(0.,-0.707106781186548,0.707106781186547));
#15130=DIRECTION('',(0.,0.707106781186547,0.707106781186548));
#15131=DIRECTION('center_axis',(0.,1.,0.));
#15132=DIRECTION('ref_axis',(1.,0.,0.));
#15133=DIRECTION('center_axis',(0.,-1.,0.));
#15134=DIRECTION('ref_axis',(1.,0.,0.));
#15135=DIRECTION('',(-0.707106781186539,0.707106781186556,8.65956056235484E-17));
#15136=DIRECTION('center_axis',(0.,1.,0.));
#15137=DIRECTION('ref_axis',(1.,0.,0.));
#15138=DIRECTION('center_axis',(0.,1.,0.));
#15139=DIRECTION('ref_axis',(0.,0.,1.));
#15140=DIRECTION('',(0.,0.,1.));
#15141=DIRECTION('',(1.,0.,0.));
#15142=DIRECTION('',(0.,0.,1.));
#15143=DIRECTION('',(1.,0.,0.));
#15144=DIRECTION('center_axis',(0.,1.,0.));
#15145=DIRECTION('ref_axis',(1.,0.,0.));
#15146=DIRECTION('center_axis',(0.,1.,0.));
#15147=DIRECTION('ref_axis',(1.,0.,0.));
#15148=DIRECTION('center_axis',(0.,1.,0.));
#15149=DIRECTION('ref_axis',(1.,0.,0.));
#15150=DIRECTION('center_axis',(0.,-1.,0.));
#15151=DIRECTION('ref_axis',(1.,0.,0.));
#15152=DIRECTION('',(0.,-1.,0.));
#15153=DIRECTION('center_axis',(0.,-1.,0.));
#15154=DIRECTION('ref_axis',(1.,0.,0.));
#15155=DIRECTION('center_axis',(0.,1.,0.));
#15156=DIRECTION('ref_axis',(1.,0.,0.));
#15157=DIRECTION('center_axis',(0.,-1.,0.));
#15158=DIRECTION('ref_axis',(1.,0.,0.));
#15159=DIRECTION('',(-0.70710678118655,0.707106781186545,8.65956056235497E-17));
#15160=DIRECTION('center_axis',(0.,-1.,0.));
#15161=DIRECTION('ref_axis',(1.,0.,0.));
#15162=DIRECTION('',(0.,-1.,0.));
#15163=DIRECTION('center_axis',(0.,-1.,0.));
#15164=DIRECTION('ref_axis',(1.,0.,0.));
#15165=DIRECTION('center_axis',(0.,1.,0.));
#15166=DIRECTION('ref_axis',(1.,0.,0.));
#15167=DIRECTION('center_axis',(0.,-1.,0.));
#15168=DIRECTION('ref_axis',(1.,0.,0.));
#15169=DIRECTION('',(-0.70710678118655,0.707106781186545,8.65956056235497E-17));
#15170=DIRECTION('center_axis',(0.,-1.,0.));
#15171=DIRECTION('ref_axis',(1.,0.,0.));
#15172=DIRECTION('',(0.,-1.,0.));
#15173=DIRECTION('center_axis',(0.,-1.,0.));
#15174=DIRECTION('ref_axis',(1.,0.,0.));
#15175=DIRECTION('center_axis',(0.,1.,0.));
#15176=DIRECTION('ref_axis',(1.,0.,0.));
#15177=DIRECTION('center_axis',(0.,-1.,0.));
#15178=DIRECTION('ref_axis',(1.,0.,0.));
#15179=DIRECTION('',(-0.707106781186539,0.707106781186556,8.65956056235484E-17));
#15180=DIRECTION('center_axis',(0.,-1.,0.));
#15181=DIRECTION('ref_axis',(1.,0.,0.));
#15182=DIRECTION('',(0.,-1.,0.));
#15183=DIRECTION('center_axis',(0.,-1.,0.));
#15184=DIRECTION('ref_axis',(1.,0.,0.));
#15185=DIRECTION('center_axis',(0.,1.,0.));
#15186=DIRECTION('ref_axis',(1.,0.,0.));
#15187=DIRECTION('center_axis',(0.,1.,0.));
#15188=DIRECTION('ref_axis',(1.,0.,0.));
#15189=DIRECTION('center_axis',(0.,1.,0.));
#15190=DIRECTION('ref_axis',(1.,0.,0.));
#15191=DIRECTION('center_axis',(0.,1.,0.));
#15192=DIRECTION('ref_axis',(1.,0.,0.));
#15193=DIRECTION('center_axis',(0.,1.,0.));
#15194=DIRECTION('ref_axis',(1.,0.,0.));
#15195=DIRECTION('center_axis',(0.,1.,0.));
#15196=DIRECTION('ref_axis',(1.,0.,0.));
#15197=DIRECTION('center_axis',(0.,1.,0.));
#15198=DIRECTION('ref_axis',(1.,0.,0.));
#15199=DIRECTION('center_axis',(0.,1.,0.));
#15200=DIRECTION('ref_axis',(1.,0.,0.));
#15201=DIRECTION('center_axis',(0.,-1.,0.));
#15202=DIRECTION('ref_axis',(1.,0.,0.));
#15203=DIRECTION('',(0.,-1.,0.));
#15204=DIRECTION('center_axis',(0.,1.,0.));
#15205=DIRECTION('ref_axis',(1.,0.,0.));
#15206=DIRECTION('center_axis',(0.,-1.,0.));
#15207=DIRECTION('ref_axis',(1.,0.,0.));
#15208=DIRECTION('',(0.,-1.,0.));
#15209=DIRECTION('center_axis',(0.,1.,0.));
#15210=DIRECTION('ref_axis',(1.,0.,0.));
#15211=DIRECTION('center_axis',(0.,-1.,0.));
#15212=DIRECTION('ref_axis',(1.,0.,0.));
#15213=DIRECTION('',(0.,-1.,0.));
#15214=DIRECTION('center_axis',(0.,1.,0.));
#15215=DIRECTION('ref_axis',(1.,0.,0.));
#15216=DIRECTION('center_axis',(0.,-1.,0.));
#15217=DIRECTION('ref_axis',(1.,0.,0.));
#15218=DIRECTION('',(0.,-1.,0.));
#15219=DIRECTION('center_axis',(0.,1.,0.));
#15220=DIRECTION('ref_axis',(1.,0.,0.));
#15221=DIRECTION('center_axis',(0.,0.707106781186548,0.707106781186548));
#15222=DIRECTION('ref_axis',(1.,0.,0.));
#15223=DIRECTION('',(0.,0.707106781186547,-0.707106781186547));
#15224=DIRECTION('',(-1.,0.,0.));
#15225=DIRECTION('',(0.,-0.707106781186547,0.707106781186547));
#15226=DIRECTION('',(1.,0.,0.));
#15227=DIRECTION('center_axis',(0.,0.,1.));
#15228=DIRECTION('ref_axis',(0.,-1.,0.));
#15229=DIRECTION('',(0.,-1.,0.));
#15230=DIRECTION('',(0.,-1.,0.));
#15231=DIRECTION('center_axis',(1.,0.,0.));
#15232=DIRECTION('ref_axis',(0.,0.,-1.));
#15233=DIRECTION('',(0.,0.,1.));
#15234=DIRECTION('',(0.,-0.707106781186548,0.707106781186547));
#15235=DIRECTION('center_axis',(1.,0.,0.));
#15236=DIRECTION('ref_axis',(0.,-0.21859823653748,0.975814947099451));
#15237=DIRECTION('',(0.,0.707106781186547,-0.707106781186547));
#15238=DIRECTION('',(0.,1.,0.));
#15239=DIRECTION('',(0.,0.707106781186549,-0.707106781186546));
#15240=DIRECTION('',(0.,0.,1.));
#15241=DIRECTION('',(0.,-0.707106781186549,-0.707106781186546));
#15242=DIRECTION('',(0.,1.,0.));
#15243=DIRECTION('',(0.,0.707106781186547,0.707106781186547));
#15244=DIRECTION('center_axis',(1.,0.,0.));
#15245=DIRECTION('ref_axis',(0.,-0.975814947099451,-0.218598236537478));
#15246=DIRECTION('',(0.,-0.707106781186548,-0.707106781186547));
#15247=DIRECTION('',(0.,0.,-1.));
#15248=DIRECTION('',(0.,0.707106781186547,0.707106781186547));
#15249=DIRECTION('',(0.,-1.,0.));
#15250=DIRECTION('center_axis',(0.,0.707106781186548,-0.707106781186548));
#15251=DIRECTION('ref_axis',(-1.,0.,0.));
#15252=DIRECTION('',(0.,-0.707106781186547,-0.707106781186547));
#15253=DIRECTION('',(-1.,0.,0.));
#15254=DIRECTION('',(1.,0.,0.));
#15255=DIRECTION('center_axis',(0.,1.,0.));
#15256=DIRECTION('ref_axis',(0.,0.,1.));
#15257=DIRECTION('',(1.,0.,0.));
#15258=DIRECTION('',(0.,0.,1.));
#15259=DIRECTION('center_axis',(0.,-0.707106781186546,0.707106781186549));
#15260=DIRECTION('ref_axis',(1.,0.,0.));
#15261=DIRECTION('',(0.,0.707106781186549,0.707106781186546));
#15262=DIRECTION('',(-1.,0.,0.));
#15263=DIRECTION('',(1.,0.,0.));
#15264=DIRECTION('center_axis',(0.,-1.,0.));
#15265=DIRECTION('ref_axis',(0.,0.,-1.));
#15266=DIRECTION('',(-1.,0.,0.));
#15267=DIRECTION('',(0.,0.,-1.));
#15268=DIRECTION('center_axis',(0.,-0.707106781186546,-0.707106781186549));
#15269=DIRECTION('ref_axis',(-1.,0.,0.));
#15270=DIRECTION('',(0.,-0.707106781186549,0.707106781186546));
#15271=DIRECTION('',(1.,0.,0.));
#15272=DIRECTION('center_axis',(1.,0.,0.));
#15273=DIRECTION('ref_axis',(0.,-0.21859823653748,0.975814947099451));
#15274=DIRECTION('',(1.,0.,0.));
#15275=DIRECTION('center_axis',(-1.,0.,0.));
#15276=DIRECTION('ref_axis',(0.,-0.21859823653748,0.975814947099451));
#15277=DIRECTION('',(1.,0.,0.));
#15278=DIRECTION('center_axis',(0.,-0.707106781186548,-0.707106781186548));
#15279=DIRECTION('ref_axis',(0.,0.707106781186548,-0.707106781186548));
#15280=DIRECTION('',(0.,0.707106781186547,-0.707106781186547));
#15281=DIRECTION('',(1.,0.,0.));
#15282=DIRECTION('center_axis',(0.,0.,-1.));
#15283=DIRECTION('ref_axis',(0.,1.,0.));
#15284=DIRECTION('',(0.,1.,0.));
#15285=DIRECTION('center_axis',(0.,0.,1.));
#15286=DIRECTION('ref_axis',(0.,-1.,0.));
#15287=DIRECTION('',(0.,-1.,0.));
#15288=DIRECTION('',(1.,0.,0.));
#15289=DIRECTION('center_axis',(0.,-0.707106781186548,0.707106781186548));
#15290=DIRECTION('ref_axis',(0.,-0.707106781186548,-0.707106781186548));
#15291=DIRECTION('',(0.,-0.707106781186547,-0.707106781186547));
#15292=DIRECTION('',(1.,0.,0.));
#15293=DIRECTION('center_axis',(1.,0.,0.));
#15294=DIRECTION('ref_axis',(0.,-0.975814947099451,-0.218598236537478));
#15295=DIRECTION('center_axis',(-1.,0.,0.));
#15296=DIRECTION('ref_axis',(0.,-0.975814947099451,-0.218598236537478));
#15297=DIRECTION('',(1.,0.,0.));
#15298=DIRECTION('center_axis',(0.,0.707106781186547,-0.707106781186548));
#15299=DIRECTION('ref_axis',(0.,0.707106781186548,0.707106781186547));
#15300=DIRECTION('',(0.,0.707106781186548,0.707106781186547));
#15301=DIRECTION('center_axis',(0.,0.,-1.));
#15302=DIRECTION('ref_axis',(0.,1.,0.));
#15303=DIRECTION('',(0.,1.,0.));
#15304=DIRECTION('center_axis',(0.,1.,0.));
#15305=DIRECTION('ref_axis',(0.,0.,1.));
#15306=DIRECTION('',(0.,0.,1.));
#15307=DIRECTION('',(1.,0.,0.));
#15308=DIRECTION('center_axis',(0.,0.707106781186547,0.707106781186548));
#15309=DIRECTION('ref_axis',(0.,-0.707106781186548,0.707106781186547));
#15310=DIRECTION('',(0.,-0.707106781186548,0.707106781186547));
#15311=DIRECTION('center_axis',(1.,0.,0.));
#15312=DIRECTION('ref_axis',(0.,0.,-1.));
#18529=CARTESIAN_POINT('',(0.,0.,0.));
#18530=CARTESIAN_POINT('Origin',(160.,0.198623766039044,-16.073623766039));
#18531=CARTESIAN_POINT('',(160.,0.,-21.8854076400856));
#18532=CARTESIAN_POINT('Origin',(160.,0.,-15.875));
#18533=CARTESIAN_POINT('',(160.,3.45131495949716,-25.3367225995828));
#18534=CARTESIAN_POINT('',(160.,-2.80658005400379,-19.0788275860818));
#18535=CARTESIAN_POINT('Origin',(160.,6.45651877953999,-22.33151877954));
#18536=CARTESIAN_POINT('Origin',(160.,6.45651877953999,-22.33151877954));
#18537=CARTESIAN_POINT('',(160.,4.61804114845495,-24.169996410625));
#18538=CARTESIAN_POINT('Origin',(160.,6.45651877953999,-22.33151877954));
#18539=CARTESIAN_POINT('Origin',(160.,12.7497691321003,-28.6247691321003));
#18540=CARTESIAN_POINT('',(160.,16.2900299668715,-35.8419852290415));
#18541=CARTESIAN_POINT('',(160.,10.9112915010153,-30.4632467631853));
#18542=CARTESIAN_POINT('',(160.,19.9669852290415,-32.1650299668715));
#18543=CARTESIAN_POINT('Ctrl Pts',(160.,19.9669852290415,-32.1650299668715));
#18544=CARTESIAN_POINT('Ctrl Pts',(159.669086687003,19.9669852290415,-32.1650299668715));
#18545=CARTESIAN_POINT('Ctrl Pts',(159.319226654958,19.8974854281187,-32.1901877843544));
#18546=CARTESIAN_POINT('Ctrl Pts',(158.680055812673,19.6321847802655,-32.3016802236596));
#18547=CARTESIAN_POINT('Ctrl Pts',(158.390338151249,19.4379182273394,-32.3893238446769));
#18548=CARTESIAN_POINT('Ctrl Pts',(157.932962788451,19.0166793035856,-32.6149113620875));
#18549=CARTESIAN_POINT('Ctrl Pts',(157.733428383838,18.7604617888226,-32.7685524550269));
#18550=CARTESIAN_POINT('Ctrl Pts',(157.466846434434,18.2360908160848,-33.1486404414343));
#18551=CARTESIAN_POINT('Ctrl Pts',(157.4,17.9686009905262,-33.3761428884047));
#18552=CARTESIAN_POINT('Ctrl Pts',(157.4,17.5011428884047,-33.8436009905262));
#18553=CARTESIAN_POINT('Ctrl Pts',(157.466846434434,17.2736404414343,-34.1110908160848));
#18554=CARTESIAN_POINT('Ctrl Pts',(157.733428383838,16.8935524550269,-34.6354617888226));
#18555=CARTESIAN_POINT('Ctrl Pts',(157.932962788451,16.7399113620875,-34.8916793035856));
#18556=CARTESIAN_POINT('Ctrl Pts',(158.390338151249,16.5143238446769,-35.3129182273394));
#18557=CARTESIAN_POINT('Ctrl Pts',(158.680055812673,16.4266802236596,-35.5071847802655));
#18558=CARTESIAN_POINT('Ctrl Pts',(159.319226654958,16.3151877843544,-35.7724854281188));
#18559=CARTESIAN_POINT('Ctrl Pts',(159.669086687003,16.2900299668715,-35.8419852290415));
#18560=CARTESIAN_POINT('Ctrl Pts',(160.,16.2900299668715,-35.8419852290415));
#18561=CARTESIAN_POINT('Ctrl Pts',(160.,16.2900299668715,-35.8419852290415));
#18562=CARTESIAN_POINT('Ctrl Pts',(160.330913312997,16.2900299668715,-35.8419852290416));
#18563=CARTESIAN_POINT('Ctrl Pts',(160.680773345042,16.3151877843544,-35.7724854281188));
#18564=CARTESIAN_POINT('Ctrl Pts',(161.319944187327,16.4266802236596,-35.5071847802655));
#18565=CARTESIAN_POINT('Ctrl Pts',(161.609661848751,16.5143238446769,-35.3129182273394));
#18566=CARTESIAN_POINT('Ctrl Pts',(162.067037211549,16.7399113620875,-34.8916793035856));
#18567=CARTESIAN_POINT('Ctrl Pts',(162.266571616162,16.8935524550269,-34.6354617888227));
#18568=CARTESIAN_POINT('Ctrl Pts',(162.533153565566,17.2736404414343,-34.1110908160848));
#18569=CARTESIAN_POINT('Ctrl Pts',(162.6,17.5011428884047,-33.8436009905262));
#18570=CARTESIAN_POINT('Ctrl Pts',(162.6,17.9686009905262,-33.3761428884047));
#18571=CARTESIAN_POINT('Ctrl Pts',(162.533153565566,18.2360908160848,-33.1486404414343));
#18572=CARTESIAN_POINT('Ctrl Pts',(162.266571616161,18.7604617888227,-32.7685524550269));
#18573=CARTESIAN_POINT('Ctrl Pts',(162.067037211549,19.0166793035856,-32.6149113620875));
#18574=CARTESIAN_POINT('Ctrl Pts',(161.609661848751,19.4379182273394,-32.3893238446769));
#18575=CARTESIAN_POINT('Ctrl Pts',(161.319944187327,19.6321847802654,-32.3016802236596));
#18576=CARTESIAN_POINT('Ctrl Pts',(160.680773345042,19.8974854281187,-32.1901877843544));
#18577=CARTESIAN_POINT('Ctrl Pts',(160.330913312997,19.9669852290415,-32.1650299668715));
#18578=CARTESIAN_POINT('Ctrl Pts',(160.,19.9669852290415,-32.1650299668715));
#18579=CARTESIAN_POINT('Origin',(90.,0.198623766039044,-16.073623766039));
#18580=CARTESIAN_POINT('',(90.,0.,-21.8854076400856));
#18581=CARTESIAN_POINT('Origin',(90.,0.,-15.875));
#18582=CARTESIAN_POINT('',(90.,3.45131495949716,-25.3367225995828));
#18583=CARTESIAN_POINT('',(90.,-2.80658005400379,-19.0788275860818));
#18584=CARTESIAN_POINT('Origin',(90.,6.45651877953999,-22.33151877954));
#18585=CARTESIAN_POINT('Origin',(90.,6.45651877953999,-22.33151877954));
#18586=CARTESIAN_POINT('',(90.,4.61804114845495,-24.169996410625));
#18587=CARTESIAN_POINT('Origin',(90.,6.45651877953999,-22.33151877954));
#18588=CARTESIAN_POINT('Origin',(90.,12.7497691321003,-28.6247691321003));
#18589=CARTESIAN_POINT('',(90.,16.2900299668715,-35.8419852290415));
#18590=CARTESIAN_POINT('',(90.,10.9112915010153,-30.4632467631853));
#18591=CARTESIAN_POINT('',(90.,19.9669852290415,-32.1650299668715));
#18592=CARTESIAN_POINT('Ctrl Pts',(90.,19.9669852290415,-32.1650299668715));
#18593=CARTESIAN_POINT('Ctrl Pts',(89.6690866870034,19.9669852290415,-32.1650299668715));
#18594=CARTESIAN_POINT('Ctrl Pts',(89.3192266549576,19.8974854281187,-32.1901877843544));
#18595=CARTESIAN_POINT('Ctrl Pts',(88.6800558126726,19.6321847802655,-32.3016802236596));
#18596=CARTESIAN_POINT('Ctrl Pts',(88.3903381512495,19.4379182273394,-32.3893238446769));
#18597=CARTESIAN_POINT('Ctrl Pts',(87.9329627884514,19.0166793035856,-32.6149113620875));
#18598=CARTESIAN_POINT('Ctrl Pts',(87.7334283838385,18.7604617888226,-32.7685524550269));
#18599=CARTESIAN_POINT('Ctrl Pts',(87.4668464344339,18.2360908160848,-33.1486404414343));
#18600=CARTESIAN_POINT('Ctrl Pts',(87.4,17.9686009905262,-33.3761428884047));
#18601=CARTESIAN_POINT('Ctrl Pts',(87.4,17.5011428884047,-33.8436009905262));
#18602=CARTESIAN_POINT('Ctrl Pts',(87.4668464344339,17.2736404414343,-34.1110908160848));
#18603=CARTESIAN_POINT('Ctrl Pts',(87.7334283838385,16.8935524550269,-34.6354617888227));
#18604=CARTESIAN_POINT('Ctrl Pts',(87.9329627884514,16.7399113620875,-34.8916793035856));
#18605=CARTESIAN_POINT('Ctrl Pts',(88.3903381512495,16.5143238446769,-35.3129182273394));
#18606=CARTESIAN_POINT('Ctrl Pts',(88.6800558126726,16.4266802236596,-35.5071847802655));
#18607=CARTESIAN_POINT('Ctrl Pts',(89.3192266549576,16.3151877843544,-35.7724854281188));
#18608=CARTESIAN_POINT('Ctrl Pts',(89.6690866870034,16.2900299668715,-35.8419852290415));
#18609=CARTESIAN_POINT('Ctrl Pts',(90.,16.2900299668715,-35.8419852290415));
#18610=CARTESIAN_POINT('Ctrl Pts',(90.,16.2900299668715,-35.8419852290415));
#18611=CARTESIAN_POINT('Ctrl Pts',(90.3309133129966,16.2900299668715,-35.8419852290415));
#18612=CARTESIAN_POINT('Ctrl Pts',(90.6807733450424,16.3151877843544,-35.7724854281188));
#18613=CARTESIAN_POINT('Ctrl Pts',(91.3199441873274,16.4266802236596,-35.5071847802655));
#18614=CARTESIAN_POINT('Ctrl Pts',(91.6096618487505,16.5143238446769,-35.3129182273394));
#18615=CARTESIAN_POINT('Ctrl Pts',(92.0670372115486,16.7399113620875,-34.8916793035856));
#18616=CARTESIAN_POINT('Ctrl Pts',(92.2665716161615,16.8935524550269,-34.6354617888227));
#18617=CARTESIAN_POINT('Ctrl Pts',(92.5331535655661,17.2736404414343,-34.1110908160848));
#18618=CARTESIAN_POINT('Ctrl Pts',(92.6,17.5011428884047,-33.8436009905262));
#18619=CARTESIAN_POINT('Ctrl Pts',(92.6,17.9686009905262,-33.3761428884047));
#18620=CARTESIAN_POINT('Ctrl Pts',(92.5331535655662,18.2360908160848,-33.1486404414343));
#18621=CARTESIAN_POINT('Ctrl Pts',(92.2665716161615,18.7604617888226,-32.7685524550269));
#18622=CARTESIAN_POINT('Ctrl Pts',(92.0670372115486,19.0166793035856,-32.6149113620875));
#18623=CARTESIAN_POINT('Ctrl Pts',(91.6096618487505,19.4379182273394,-32.3893238446769));
#18624=CARTESIAN_POINT('Ctrl Pts',(91.3199441873274,19.6321847802655,-32.3016802236596));
#18625=CARTESIAN_POINT('Ctrl Pts',(90.6807733450424,19.8974854281187,-32.1901877843544));
#18626=CARTESIAN_POINT('Ctrl Pts',(90.3309133129966,19.9669852290415,-32.1650299668715));
#18627=CARTESIAN_POINT('Ctrl Pts',(90.,19.9669852290415,-32.1650299668715));
#18628=CARTESIAN_POINT('Origin',(20.,0.198623766039044,-16.073623766039));
#18629=CARTESIAN_POINT('',(20.,0.,-21.8854076400856));
#18630=CARTESIAN_POINT('Origin',(20.,0.,-15.875));
#18631=CARTESIAN_POINT('',(20.,3.45131495949716,-25.3367225995828));
#18632=CARTESIAN_POINT('',(20.,-2.80658005400379,-19.0788275860818));
#18633=CARTESIAN_POINT('Origin',(20.,6.45651877953999,-22.33151877954));
#18634=CARTESIAN_POINT('Origin',(20.,6.45651877953999,-22.33151877954));
#18635=CARTESIAN_POINT('',(20.,4.61804114845495,-24.169996410625));
#18636=CARTESIAN_POINT('Origin',(20.,6.45651877953999,-22.33151877954));
#18637=CARTESIAN_POINT('Origin',(20.,12.7497691321003,-28.6247691321003));
#18638=CARTESIAN_POINT('',(20.,16.2900299668715,-35.8419852290415));
#18639=CARTESIAN_POINT('',(20.,10.9112915010153,-30.4632467631853));
#18640=CARTESIAN_POINT('',(20.,19.9669852290415,-32.1650299668715));
#18641=CARTESIAN_POINT('Ctrl Pts',(20.,19.9669852290415,-32.1650299668715));
#18642=CARTESIAN_POINT('Ctrl Pts',(19.6690866870034,19.9669852290415,-32.1650299668715));
#18643=CARTESIAN_POINT('Ctrl Pts',(19.3192266549576,19.8974854281187,-32.1901877843544));
#18644=CARTESIAN_POINT('Ctrl Pts',(18.6800558126726,19.6321847802655,-32.3016802236596));
#18645=CARTESIAN_POINT('Ctrl Pts',(18.3903381512495,19.4379182273394,-32.3893238446769));
#18646=CARTESIAN_POINT('Ctrl Pts',(17.9329627884514,19.0166793035856,-32.6149113620875));
#18647=CARTESIAN_POINT('Ctrl Pts',(17.7334283838385,18.7604617888226,-32.7685524550269));
#18648=CARTESIAN_POINT('Ctrl Pts',(17.4668464344338,18.2360908160848,-33.1486404414343));
#18649=CARTESIAN_POINT('Ctrl Pts',(17.4,17.9686009905262,-33.3761428884047));
#18650=CARTESIAN_POINT('Ctrl Pts',(17.4,17.5011428884047,-33.8436009905262));
#18651=CARTESIAN_POINT('Ctrl Pts',(17.4668464344338,17.2736404414343,-34.1110908160848));
#18652=CARTESIAN_POINT('Ctrl Pts',(17.7334283838385,16.8935524550269,-34.6354617888227));
#18653=CARTESIAN_POINT('Ctrl Pts',(17.9329627884514,16.7399113620875,-34.8916793035856));
#18654=CARTESIAN_POINT('Ctrl Pts',(18.3903381512495,16.5143238446769,-35.3129182273394));
#18655=CARTESIAN_POINT('Ctrl Pts',(18.6800558126726,16.4266802236596,-35.5071847802655));
#18656=CARTESIAN_POINT('Ctrl Pts',(19.3192266549576,16.3151877843544,-35.7724854281188));
#18657=CARTESIAN_POINT('Ctrl Pts',(19.6690866870034,16.2900299668715,-35.8419852290415));
#18658=CARTESIAN_POINT('Ctrl Pts',(20.,16.2900299668715,-35.8419852290415));
#18659=CARTESIAN_POINT('Ctrl Pts',(20.,16.2900299668715,-35.8419852290415));
#18660=CARTESIAN_POINT('Ctrl Pts',(20.3309133129966,16.2900299668715,-35.8419852290415));
#18661=CARTESIAN_POINT('Ctrl Pts',(20.6807733450423,16.3151877843544,-35.7724854281188));
#18662=CARTESIAN_POINT('Ctrl Pts',(21.3199441873274,16.4266802236596,-35.5071847802655));
#18663=CARTESIAN_POINT('Ctrl Pts',(21.6096618487505,16.5143238446769,-35.3129182273394));
#18664=CARTESIAN_POINT('Ctrl Pts',(22.0670372115486,16.7399113620875,-34.8916793035856));
#18665=CARTESIAN_POINT('Ctrl Pts',(22.2665716161615,16.8935524550269,-34.6354617888227));
#18666=CARTESIAN_POINT('Ctrl Pts',(22.5331535655662,17.2736404414343,-34.1110908160848));
#18667=CARTESIAN_POINT('Ctrl Pts',(22.6,17.5011428884047,-33.8436009905262));
#18668=CARTESIAN_POINT('Ctrl Pts',(22.6,17.9686009905262,-33.3761428884047));
#18669=CARTESIAN_POINT('Ctrl Pts',(22.5331535655662,18.2360908160848,-33.1486404414343));
#18670=CARTESIAN_POINT('Ctrl Pts',(22.2665716161615,18.7604617888226,-32.7685524550269));
#18671=CARTESIAN_POINT('Ctrl Pts',(22.0670372115486,19.0166793035856,-32.6149113620875));
#18672=CARTESIAN_POINT('Ctrl Pts',(21.6096618487505,19.4379182273394,-32.3893238446769));
#18673=CARTESIAN_POINT('Ctrl Pts',(21.3199441873274,19.6321847802655,-32.3016802236596));
#18674=CARTESIAN_POINT('Ctrl Pts',(20.6807733450424,19.8974854281187,-32.1901877843544));
#18675=CARTESIAN_POINT('Ctrl Pts',(20.3309133129966,19.9669852290415,-32.1650299668715));
#18676=CARTESIAN_POINT('Ctrl Pts',(20.,19.9669852290415,-32.1650299668715));
#18677=CARTESIAN_POINT('Origin',(160.,0.198623766039043,16.073623766039));
#18678=CARTESIAN_POINT('',(160.,0.,9.86459235991433));
#18679=CARTESIAN_POINT('Origin',(160.,0.,15.875));
#18680=CARTESIAN_POINT('',(160.,9.46172259958282,19.3263149594972));
#18681=CARTESIAN_POINT('',(160.,3.20382758608187,13.0684199459962));
#18682=CARTESIAN_POINT('Origin',(160.,6.45651877953999,22.33151877954));
#18683=CARTESIAN_POINT('Origin',(160.,6.45651877953999,22.33151877954));
#18684=CARTESIAN_POINT('',(160.,8.29499641062501,20.4930411484549));
#18685=CARTESIAN_POINT('Origin',(160.,6.45651877953999,22.33151877954));
#18686=CARTESIAN_POINT('Origin',(160.,12.7497691321003,28.6247691321003));
#18687=CARTESIAN_POINT('',(160.,19.9669852290415,32.1650299668715));
#18688=CARTESIAN_POINT('',(160.,14.5882467631853,26.7862915010153));
#18689=CARTESIAN_POINT('',(160.,16.2900299668715,35.8419852290415));
#18690=CARTESIAN_POINT('Ctrl Pts',(160.,16.2900299668715,35.8419852290415));
#18691=CARTESIAN_POINT('Ctrl Pts',(159.669086687003,16.2900299668715,35.8419852290415));
#18692=CARTESIAN_POINT('Ctrl Pts',(159.319226654958,16.3151877843544,35.7724854281188));
#18693=CARTESIAN_POINT('Ctrl Pts',(158.680055812673,16.4266802236596,35.5071847802655));
#18694=CARTESIAN_POINT('Ctrl Pts',(158.390338151249,16.5143238446769,35.3129182273394));
#18695=CARTESIAN_POINT('Ctrl Pts',(157.932962788451,16.7399113620875,34.8916793035856));
#18696=CARTESIAN_POINT('Ctrl Pts',(157.733428383838,16.8935524550269,34.6354617888226));
#18697=CARTESIAN_POINT('Ctrl Pts',(157.466846434434,17.2736404414343,34.1110908160848));
#18698=CARTESIAN_POINT('Ctrl Pts',(157.4,17.5011428884047,33.8436009905262));
#18699=CARTESIAN_POINT('Ctrl Pts',(157.4,17.9686009905262,33.3761428884047));
#18700=CARTESIAN_POINT('Ctrl Pts',(157.466846434434,18.2360908160848,33.1486404414343));
#18701=CARTESIAN_POINT('Ctrl Pts',(157.733428383838,18.7604617888226,32.7685524550269));
#18702=CARTESIAN_POINT('Ctrl Pts',(157.932962788451,19.0166793035856,32.6149113620875));
#18703=CARTESIAN_POINT('Ctrl Pts',(158.390338151249,19.4379182273394,32.3893238446769));
#18704=CARTESIAN_POINT('Ctrl Pts',(158.680055812673,19.6321847802654,32.3016802236596));
#18705=CARTESIAN_POINT('Ctrl Pts',(159.319226654958,19.8974854281187,32.1901877843544));
#18706=CARTESIAN_POINT('Ctrl Pts',(159.669086687003,19.9669852290415,32.1650299668715));
#18707=CARTESIAN_POINT('Ctrl Pts',(160.,19.9669852290415,32.1650299668715));
#18708=CARTESIAN_POINT('Ctrl Pts',(160.,19.9669852290415,32.1650299668715));
#18709=CARTESIAN_POINT('Ctrl Pts',(160.330913312997,19.9669852290415,32.1650299668715));
#18710=CARTESIAN_POINT('Ctrl Pts',(160.680773345042,19.8974854281187,32.1901877843544));
#18711=CARTESIAN_POINT('Ctrl Pts',(161.319944187327,19.6321847802655,32.3016802236596));
#18712=CARTESIAN_POINT('Ctrl Pts',(161.609661848751,19.4379182273394,32.3893238446769));
#18713=CARTESIAN_POINT('Ctrl Pts',(162.067037211549,19.0166793035856,32.6149113620875));
#18714=CARTESIAN_POINT('Ctrl Pts',(162.266571616162,18.7604617888227,32.7685524550269));
#18715=CARTESIAN_POINT('Ctrl Pts',(162.533153565566,18.2360908160848,33.1486404414343));
#18716=CARTESIAN_POINT('Ctrl Pts',(162.6,17.9686009905262,33.3761428884047));
#18717=CARTESIAN_POINT('Ctrl Pts',(162.6,17.5011428884047,33.8436009905262));
#18718=CARTESIAN_POINT('Ctrl Pts',(162.533153565566,17.2736404414343,34.1110908160848));
#18719=CARTESIAN_POINT('Ctrl Pts',(162.266571616161,16.8935524550269,34.6354617888227));
#18720=CARTESIAN_POINT('Ctrl Pts',(162.067037211549,16.7399113620875,34.8916793035856));
#18721=CARTESIAN_POINT('Ctrl Pts',(161.609661848751,16.5143238446769,35.3129182273394));
#18722=CARTESIAN_POINT('Ctrl Pts',(161.319944187327,16.4266802236596,35.5071847802655));
#18723=CARTESIAN_POINT('Ctrl Pts',(160.680773345042,16.3151877843544,35.7724854281188));
#18724=CARTESIAN_POINT('Ctrl Pts',(160.330913312997,16.2900299668715,35.8419852290415));
#18725=CARTESIAN_POINT('Ctrl Pts',(160.,16.2900299668715,35.8419852290415));
#18726=CARTESIAN_POINT('Origin',(90.,0.198623766039043,16.073623766039));
#18727=CARTESIAN_POINT('',(90.,0.,9.86459235991433));
#18728=CARTESIAN_POINT('Origin',(90.,0.,15.875));
#18729=CARTESIAN_POINT('',(90.,9.46172259958282,19.3263149594972));
#18730=CARTESIAN_POINT('',(90.,3.20382758608187,13.0684199459962));
#18731=CARTESIAN_POINT('Origin',(90.,6.45651877953999,22.33151877954));
#18732=CARTESIAN_POINT('Origin',(90.,6.45651877953999,22.33151877954));
#18733=CARTESIAN_POINT('',(90.,8.29499641062501,20.4930411484549));
#18734=CARTESIAN_POINT('Origin',(90.,6.45651877953999,22.33151877954));
#18735=CARTESIAN_POINT('Origin',(90.,12.7497691321003,28.6247691321003));
#18736=CARTESIAN_POINT('',(90.,19.9669852290415,32.1650299668715));
#18737=CARTESIAN_POINT('',(90.,14.5882467631853,26.7862915010153));
#18738=CARTESIAN_POINT('',(90.,16.2900299668715,35.8419852290415));
#18739=CARTESIAN_POINT('Ctrl Pts',(90.,16.2900299668715,35.8419852290415));
#18740=CARTESIAN_POINT('Ctrl Pts',(89.6690866870034,16.2900299668715,35.8419852290415));
#18741=CARTESIAN_POINT('Ctrl Pts',(89.3192266549576,16.3151877843544,35.7724854281188));
#18742=CARTESIAN_POINT('Ctrl Pts',(88.6800558126726,16.4266802236596,35.5071847802655));
#18743=CARTESIAN_POINT('Ctrl Pts',(88.3903381512495,16.5143238446769,35.3129182273394));
#18744=CARTESIAN_POINT('Ctrl Pts',(87.9329627884514,16.7399113620875,34.8916793035856));
#18745=CARTESIAN_POINT('Ctrl Pts',(87.7334283838385,16.8935524550269,34.6354617888227));
#18746=CARTESIAN_POINT('Ctrl Pts',(87.4668464344339,17.2736404414343,34.1110908160848));
#18747=CARTESIAN_POINT('Ctrl Pts',(87.4,17.5011428884047,33.8436009905262));
#18748=CARTESIAN_POINT('Ctrl Pts',(87.4,17.9686009905262,33.3761428884047));
#18749=CARTESIAN_POINT('Ctrl Pts',(87.4668464344339,18.2360908160848,33.1486404414343));
#18750=CARTESIAN_POINT('Ctrl Pts',(87.7334283838385,18.7604617888226,32.7685524550269));
#18751=CARTESIAN_POINT('Ctrl Pts',(87.9329627884514,19.0166793035856,32.6149113620875));
#18752=CARTESIAN_POINT('Ctrl Pts',(88.3903381512495,19.4379182273394,32.3893238446769));
#18753=CARTESIAN_POINT('Ctrl Pts',(88.6800558126726,19.6321847802655,32.3016802236596));
#18754=CARTESIAN_POINT('Ctrl Pts',(89.3192266549576,19.8974854281187,32.1901877843544));
#18755=CARTESIAN_POINT('Ctrl Pts',(89.6690866870034,19.9669852290415,32.1650299668715));
#18756=CARTESIAN_POINT('Ctrl Pts',(90.,19.9669852290415,32.1650299668715));
#18757=CARTESIAN_POINT('Ctrl Pts',(90.,19.9669852290415,32.1650299668715));
#18758=CARTESIAN_POINT('Ctrl Pts',(90.3309133129966,19.9669852290415,32.1650299668715));
#18759=CARTESIAN_POINT('Ctrl Pts',(90.6807733450424,19.8974854281188,32.1901877843544));
#18760=CARTESIAN_POINT('Ctrl Pts',(91.3199441873274,19.6321847802655,32.3016802236596));
#18761=CARTESIAN_POINT('Ctrl Pts',(91.6096618487505,19.4379182273394,32.3893238446769));
#18762=CARTESIAN_POINT('Ctrl Pts',(92.0670372115486,19.0166793035856,32.6149113620875));
#18763=CARTESIAN_POINT('Ctrl Pts',(92.2665716161615,18.7604617888226,32.7685524550269));
#18764=CARTESIAN_POINT('Ctrl Pts',(92.5331535655662,18.2360908160848,33.1486404414343));
#18765=CARTESIAN_POINT('Ctrl Pts',(92.6,17.9686009905262,33.3761428884047));
#18766=CARTESIAN_POINT('Ctrl Pts',(92.6,17.5011428884047,33.8436009905262));
#18767=CARTESIAN_POINT('Ctrl Pts',(92.5331535655661,17.2736404414343,34.1110908160848));
#18768=CARTESIAN_POINT('Ctrl Pts',(92.2665716161615,16.8935524550269,34.6354617888227));
#18769=CARTESIAN_POINT('Ctrl Pts',(92.0670372115486,16.7399113620875,34.8916793035856));
#18770=CARTESIAN_POINT('Ctrl Pts',(91.6096618487505,16.5143238446769,35.3129182273394));
#18771=CARTESIAN_POINT('Ctrl Pts',(91.3199441873274,16.4266802236596,35.5071847802655));
#18772=CARTESIAN_POINT('Ctrl Pts',(90.6807733450424,16.3151877843544,35.7724854281188));
#18773=CARTESIAN_POINT('Ctrl Pts',(90.3309133129966,16.2900299668715,35.8419852290415));
#18774=CARTESIAN_POINT('Ctrl Pts',(90.,16.2900299668715,35.8419852290415));
#18775=CARTESIAN_POINT('Origin',(20.,0.198623766039043,16.073623766039));
#18776=CARTESIAN_POINT('',(20.,0.,9.86459235991433));
#18777=CARTESIAN_POINT('Origin',(20.,0.,15.875));
#18778=CARTESIAN_POINT('',(20.,9.46172259958282,19.3263149594972));
#18779=CARTESIAN_POINT('',(20.,3.20382758608187,13.0684199459962));
#18780=CARTESIAN_POINT('Origin',(20.,6.45651877953999,22.33151877954));
#18781=CARTESIAN_POINT('Origin',(20.,6.45651877953999,22.33151877954));
#18782=CARTESIAN_POINT('',(20.,8.29499641062501,20.4930411484549));
#18783=CARTESIAN_POINT('Origin',(20.,6.45651877953999,22.33151877954));
#18784=CARTESIAN_POINT('Origin',(20.,12.7497691321003,28.6247691321003));
#18785=CARTESIAN_POINT('',(20.,19.9669852290415,32.1650299668715));
#18786=CARTESIAN_POINT('',(20.,14.5882467631853,26.7862915010153));
#18787=CARTESIAN_POINT('',(20.,16.2900299668715,35.8419852290415));
#18788=CARTESIAN_POINT('Ctrl Pts',(20.,16.2900299668715,35.8419852290415));
#18789=CARTESIAN_POINT('Ctrl Pts',(19.6690866870034,16.2900299668715,35.8419852290415));
#18790=CARTESIAN_POINT('Ctrl Pts',(19.3192266549576,16.3151877843544,35.7724854281188));
#18791=CARTESIAN_POINT('Ctrl Pts',(18.6800558126726,16.4266802236596,35.5071847802655));
#18792=CARTESIAN_POINT('Ctrl Pts',(18.3903381512495,16.5143238446769,35.3129182273394));
#18793=CARTESIAN_POINT('Ctrl Pts',(17.9329627884514,16.7399113620875,34.8916793035856));
#18794=CARTESIAN_POINT('Ctrl Pts',(17.7334283838385,16.8935524550269,34.6354617888227));
#18795=CARTESIAN_POINT('Ctrl Pts',(17.4668464344338,17.2736404414343,34.1110908160848));
#18796=CARTESIAN_POINT('Ctrl Pts',(17.4,17.5011428884047,33.8436009905262));
#18797=CARTESIAN_POINT('Ctrl Pts',(17.4,17.9686009905262,33.3761428884047));
#18798=CARTESIAN_POINT('Ctrl Pts',(17.4668464344338,18.2360908160848,33.1486404414343));
#18799=CARTESIAN_POINT('Ctrl Pts',(17.7334283838385,18.7604617888226,32.7685524550269));
#18800=CARTESIAN_POINT('Ctrl Pts',(17.9329627884514,19.0166793035856,32.6149113620875));
#18801=CARTESIAN_POINT('Ctrl Pts',(18.3903381512495,19.4379182273394,32.3893238446769));
#18802=CARTESIAN_POINT('Ctrl Pts',(18.6800558126726,19.6321847802655,32.3016802236596));
#18803=CARTESIAN_POINT('Ctrl Pts',(19.3192266549576,19.8974854281187,32.1901877843544));
#18804=CARTESIAN_POINT('Ctrl Pts',(19.6690866870034,19.9669852290415,32.1650299668715));
#18805=CARTESIAN_POINT('Ctrl Pts',(20.,19.9669852290415,32.1650299668715));
#18806=CARTESIAN_POINT('Ctrl Pts',(20.,19.9669852290415,32.1650299668715));
#18807=CARTESIAN_POINT('Ctrl Pts',(20.3309133129966,19.9669852290415,32.1650299668715));
#18808=CARTESIAN_POINT('Ctrl Pts',(20.6807733450423,19.8974854281188,32.1901877843544));
#18809=CARTESIAN_POINT('Ctrl Pts',(21.3199441873274,19.6321847802655,32.3016802236596));
#18810=CARTESIAN_POINT('Ctrl Pts',(21.6096618487505,19.4379182273394,32.3893238446769));
#18811=CARTESIAN_POINT('Ctrl Pts',(22.0670372115486,19.0166793035856,32.6149113620875));
#18812=CARTESIAN_POINT('Ctrl Pts',(22.2665716161615,18.7604617888226,32.7685524550269));
#18813=CARTESIAN_POINT('Ctrl Pts',(22.5331535655662,18.2360908160848,33.1486404414343));
#18814=CARTESIAN_POINT('Ctrl Pts',(22.6,17.9686009905262,33.3761428884047));
#18815=CARTESIAN_POINT('Ctrl Pts',(22.6,17.5011428884047,33.8436009905262));
#18816=CARTESIAN_POINT('Ctrl Pts',(22.5331535655662,17.2736404414343,34.1110908160848));
#18817=CARTESIAN_POINT('Ctrl Pts',(22.2665716161615,16.8935524550269,34.6354617888227));
#18818=CARTESIAN_POINT('Ctrl Pts',(22.0670372115486,16.7399113620875,34.8916793035856));
#18819=CARTESIAN_POINT('Ctrl Pts',(21.6096618487505,16.5143238446769,35.3129182273394));
#18820=CARTESIAN_POINT('Ctrl Pts',(21.3199441873274,16.4266802236596,35.5071847802655));
#18821=CARTESIAN_POINT('Ctrl Pts',(20.6807733450423,16.3151877843544,35.7724854281188));
#18822=CARTESIAN_POINT('Ctrl Pts',(20.3309133129966,16.2900299668715,35.8419852290415));
#18823=CARTESIAN_POINT('Ctrl Pts',(20.,16.2900299668715,35.8419852290415));
#18824=CARTESIAN_POINT('Origin',(140.8,12.35,9.525));
#18825=CARTESIAN_POINT('',(135.45,12.2,9.525));
#18826=CARTESIAN_POINT('Origin',(140.8,12.2,9.525));
#18827=CARTESIAN_POINT('',(135.15,12.5,9.525));
#18828=CARTESIAN_POINT('',(135.3,12.35,9.525));
#18829=CARTESIAN_POINT('Origin',(140.8,12.5,9.525));
#18830=CARTESIAN_POINT('Origin',(0.,12.5,-15.875));
#18831=CARTESIAN_POINT('',(0.,12.5,-15.875));
#18832=CARTESIAN_POINT('',(0.,12.5,15.875));
#18833=CARTESIAN_POINT('',(0.,12.5,-15.875));
#18834=CARTESIAN_POINT('',(180.,12.5,15.875));
#18835=CARTESIAN_POINT('',(0.,12.5,15.875));
#18836=CARTESIAN_POINT('',(180.,12.5,-15.875));
#18837=CARTESIAN_POINT('',(180.,12.5,-15.875));
#18838=CARTESIAN_POINT('',(0.,12.5,-15.875));
#18839=CARTESIAN_POINT('',(33.55,12.5,-9.525));
#18840=CARTESIAN_POINT('Origin',(39.2,12.5,-9.525));
#18841=CARTESIAN_POINT('',(135.15,12.5,-9.525));
#18842=CARTESIAN_POINT('Origin',(140.8,12.5,-9.525));
#18843=CARTESIAN_POINT('',(33.55,12.5,9.525));
#18844=CARTESIAN_POINT('Origin',(39.2,12.5,9.525));
#18845=CARTESIAN_POINT('Origin',(140.8,12.5,9.525));
#18846=CARTESIAN_POINT('',(135.45,5.9,9.525));
#18847=CARTESIAN_POINT('',(135.45,12.5,9.525));
#18848=CARTESIAN_POINT('Origin',(140.8,5.9,9.525));
#18849=CARTESIAN_POINT('Origin',(39.2,12.35,-9.525));
#18850=CARTESIAN_POINT('',(33.85,12.2,-9.525));
#18851=CARTESIAN_POINT('Origin',(39.2,12.2,-9.525));
#18852=CARTESIAN_POINT('',(33.7,12.35,-9.525));
#18853=CARTESIAN_POINT('Origin',(39.2,12.5,-9.525));
#18854=CARTESIAN_POINT('',(33.85,5.9,-9.525));
#18855=CARTESIAN_POINT('',(33.85,12.5,-9.525));
#18856=CARTESIAN_POINT('Origin',(39.2,5.9,-9.525));
#18857=CARTESIAN_POINT('Origin',(39.2,12.35,9.525));
#18858=CARTESIAN_POINT('',(33.85,12.2,9.525));
#18859=CARTESIAN_POINT('Origin',(39.2,12.2,9.525));
#18860=CARTESIAN_POINT('',(33.7,12.35,9.525));
#18861=CARTESIAN_POINT('Origin',(39.2,12.5,9.525));
#18862=CARTESIAN_POINT('',(33.85,5.9,9.525));
#18863=CARTESIAN_POINT('',(33.85,12.5,9.525));
#18864=CARTESIAN_POINT('Origin',(39.2,5.9,9.525));
#18865=CARTESIAN_POINT('Origin',(140.8,12.35,-9.525));
#18866=CARTESIAN_POINT('',(135.45,12.2,-9.525));
#18867=CARTESIAN_POINT('Origin',(140.8,12.2,-9.525));
#18868=CARTESIAN_POINT('',(135.3,12.35,-9.525));
#18869=CARTESIAN_POINT('Origin',(140.8,12.5,-9.525));
#18870=CARTESIAN_POINT('',(135.45,5.9,-9.525));
#18871=CARTESIAN_POINT('',(135.45,12.5,-9.525));
#18872=CARTESIAN_POINT('Origin',(140.8,5.9,-9.525));
#18873=CARTESIAN_POINT('Origin',(140.8,5.9,-9.525));
#18874=CARTESIAN_POINT('',(137.244,5.9,-9.525));
#18875=CARTESIAN_POINT('Origin',(140.8,5.9,-9.525));
#18876=CARTESIAN_POINT('Origin',(39.2,5.9,9.525));
#18877=CARTESIAN_POINT('',(35.644,5.9,9.525));
#18878=CARTESIAN_POINT('Origin',(39.2,5.9,9.525));
#18879=CARTESIAN_POINT('Origin',(39.2,5.9,-9.525));
#18880=CARTESIAN_POINT('',(35.644,5.9,-9.525));
#18881=CARTESIAN_POINT('Origin',(39.2,5.9,-9.525));
#18882=CARTESIAN_POINT('Origin',(140.8,5.9,9.525));
#18883=CARTESIAN_POINT('',(137.244,5.9,9.525));
#18884=CARTESIAN_POINT('Origin',(140.8,5.9,9.525));
#18885=CARTESIAN_POINT('Origin',(140.8,12.5,-9.525));
#18886=CARTESIAN_POINT('',(137.244,0.,-9.525));
#18887=CARTESIAN_POINT('',(137.244,12.5,-9.525));
#18888=CARTESIAN_POINT('Origin',(140.8,0.,-9.525));
#18889=CARTESIAN_POINT('Origin',(39.2,12.5,9.525));
#18890=CARTESIAN_POINT('',(35.644,0.,9.525));
#18891=CARTESIAN_POINT('',(35.644,12.5,9.525));
#18892=CARTESIAN_POINT('Origin',(39.2,0.,9.525));
#18893=CARTESIAN_POINT('Origin',(39.2,12.5,-9.525));
#18894=CARTESIAN_POINT('',(35.644,0.,-9.525));
#18895=CARTESIAN_POINT('',(35.644,12.5,-9.525));
#18896=CARTESIAN_POINT('Origin',(39.2,0.,-9.525));
#18897=CARTESIAN_POINT('Origin',(140.8,12.5,9.525));
#18898=CARTESIAN_POINT('',(137.244,0.,9.525));
#18899=CARTESIAN_POINT('',(137.244,12.5,9.525));
#18900=CARTESIAN_POINT('Origin',(140.8,0.,9.525));
#18901=CARTESIAN_POINT('Origin',(0.,17.3,-16.075));
#18902=CARTESIAN_POINT('',(180.,17.1,-15.875));
#18903=CARTESIAN_POINT('',(180.,17.5,-16.275));
#18904=CARTESIAN_POINT('',(180.,11.5608626497484,-10.3358626497484));
#18905=CARTESIAN_POINT('',(0.,17.5,-16.275));
#18906=CARTESIAN_POINT('',(0.,17.5,-16.275));
#18907=CARTESIAN_POINT('',(0.,17.1,-15.875));
#18908=CARTESIAN_POINT('',(0.,11.5608626497484,-10.3358626497484));
#18909=CARTESIAN_POINT('',(0.,17.1,-15.875));
#18910=CARTESIAN_POINT('Origin',(0.,17.5,-15.875));
#18911=CARTESIAN_POINT('',(0.,17.5,-15.875));
#18912=CARTESIAN_POINT('',(180.,17.5,-15.875));
#18913=CARTESIAN_POINT('Origin',(0.,10.4184505989935,0.));
#18914=CARTESIAN_POINT('',(0.,17.5,-28.5666738879315));
#18915=CARTESIAN_POINT('',(0.,17.5,-28.5666738879315));
#18916=CARTESIAN_POINT('',(0.,20.836901197987,-31.9035750859185));
#18917=CARTESIAN_POINT('',(0.,20.836901197987,-31.9035750859185));
#18918=CARTESIAN_POINT('',(0.,16.0285750859185,-36.711901197987));
#18919=CARTESIAN_POINT('Origin',(0.,22.225,-38.1));
#18920=CARTESIAN_POINT('',(0.,4.71667388793148,-25.4));
#18921=CARTESIAN_POINT('',(0.,4.71667388793148,-25.4));
#18922=CARTESIAN_POINT('',(0.,0.5,-25.4));
#18923=CARTESIAN_POINT('',(0.,0.,-25.4));
#18924=CARTESIAN_POINT('',(0.,0.,-24.9));
#18925=CARTESIAN_POINT('',(0.,-3.49538735025162,-21.4046126497484));
#18926=CARTESIAN_POINT('',(0.,0.,24.9));
#18927=CARTESIAN_POINT('',(0.,0.,0.));
#18928=CARTESIAN_POINT('',(0.,0.5,25.4));
#18929=CARTESIAN_POINT('',(0.,-3.49538735025162,21.4046126497484));
#18930=CARTESIAN_POINT('',(0.,4.71667388793148,25.4));
#18931=CARTESIAN_POINT('',(0.,0.,25.4));
#18932=CARTESIAN_POINT('',(0.,16.0285750859185,36.711901197987));
#18933=CARTESIAN_POINT('',(0.,4.71667388793148,25.4));
#18934=CARTESIAN_POINT('',(0.,20.836901197987,31.9035750859185));
#18935=CARTESIAN_POINT('Origin',(0.,22.225,38.1));
#18936=CARTESIAN_POINT('',(0.,17.5,28.5666738879315));
#18937=CARTESIAN_POINT('',(0.,20.836901197987,31.9035750859185));
#18938=CARTESIAN_POINT('',(0.,17.5,16.275));
#18939=CARTESIAN_POINT('',(0.,17.5,28.5666738879315));
#18940=CARTESIAN_POINT('',(0.,17.1,15.875));
#18941=CARTESIAN_POINT('',(0.,11.5608626497484,10.3358626497484));
#18942=CARTESIAN_POINT('',(0.,17.5,15.875));
#18943=CARTESIAN_POINT('Origin',(0.,17.3,16.075));
#18944=CARTESIAN_POINT('',(180.,17.5,16.275));
#18945=CARTESIAN_POINT('',(180.,17.1,15.875));
#18946=CARTESIAN_POINT('',(180.,11.5608626497484,10.3358626497484));
#18947=CARTESIAN_POINT('',(0.,17.1,15.875));
#18948=CARTESIAN_POINT('',(0.,17.5,16.275));
#18949=CARTESIAN_POINT('Origin',(0.,17.5,15.875));
#18950=CARTESIAN_POINT('',(180.,17.5,28.5666738879315));
#18951=CARTESIAN_POINT('',(0.,17.5,28.5666738879315));
#18952=CARTESIAN_POINT('',(180.,17.5,28.5666738879315));
#18953=CARTESIAN_POINT('Origin',(0.,0.25,25.15));
#18954=CARTESIAN_POINT('',(180.,0.,24.9));
#18955=CARTESIAN_POINT('',(180.,0.5,25.4));
#18956=CARTESIAN_POINT('',(180.,-3.49538735025162,21.4046126497484));
#18957=CARTESIAN_POINT('',(0.,0.5,25.4));
#18958=CARTESIAN_POINT('',(0.,0.,24.9));
#18959=CARTESIAN_POINT('Origin',(0.,0.,25.4));
#18960=CARTESIAN_POINT('',(180.,0.,-24.9));
#18961=CARTESIAN_POINT('',(0.,0.,-24.9));
#18962=CARTESIAN_POINT('',(180.,0.,0.));
#18963=CARTESIAN_POINT('Origin',(0.,0.25,-25.15));
#18964=CARTESIAN_POINT('',(180.,0.5,-25.4));
#18965=CARTESIAN_POINT('',(180.,-3.49538735025162,-21.4046126497484));
#18966=CARTESIAN_POINT('',(0.,0.5,-25.4));
#18967=CARTESIAN_POINT('Origin',(0.,22.225,-38.1));
#18968=CARTESIAN_POINT('',(180.,20.836901197987,-31.9035750859185));
#18969=CARTESIAN_POINT('',(0.,20.836901197987,-31.9035750859185));
#18970=CARTESIAN_POINT('',(180.,16.0285750859185,-36.711901197987));
#18971=CARTESIAN_POINT('Origin',(180.,22.225,-38.1));
#18972=CARTESIAN_POINT('',(0.,16.0285750859185,-36.711901197987));
#18973=CARTESIAN_POINT('Origin',(0.,4.71667388793148,-25.4));
#18974=CARTESIAN_POINT('',(180.,4.71667388793148,-25.4));
#18975=CARTESIAN_POINT('',(180.,4.71667388793148,-25.4));
#18976=CARTESIAN_POINT('',(0.,4.71667388793148,-25.4));
#18977=CARTESIAN_POINT('Origin',(0.,0.,-25.4));
#18978=CARTESIAN_POINT('',(180.,0.,-25.4));
#18979=CARTESIAN_POINT('Origin',(0.,4.71667388793148,25.4));
#18980=CARTESIAN_POINT('',(180.,4.71667388793148,25.4));
#18981=CARTESIAN_POINT('',(180.,0.,25.4));
#18982=CARTESIAN_POINT('',(0.,4.71667388793148,25.4));
#18983=CARTESIAN_POINT('Origin',(0.,16.0285750859185,36.711901197987));
#18984=CARTESIAN_POINT('',(180.,16.0285750859185,36.711901197987));
#18985=CARTESIAN_POINT('',(180.,4.71667388793148,25.4));
#18986=CARTESIAN_POINT('',(0.,16.0285750859185,36.711901197987));
#18987=CARTESIAN_POINT('Origin',(0.,22.225,38.1));
#18988=CARTESIAN_POINT('',(180.,20.836901197987,31.9035750859185));
#18989=CARTESIAN_POINT('Origin',(180.,22.225,38.1));
#18990=CARTESIAN_POINT('',(0.,20.836901197987,31.9035750859185));
#18991=CARTESIAN_POINT('Origin',(0.,17.5,28.5666738879315));
#18992=CARTESIAN_POINT('',(180.,20.836901197987,31.9035750859185));
#18993=CARTESIAN_POINT('Origin',(0.,12.5,15.875));
#18994=CARTESIAN_POINT('',(180.,17.5,15.875));
#18995=CARTESIAN_POINT('Origin',(0.,17.5,-28.5666738879315));
#18996=CARTESIAN_POINT('',(180.,17.5,-28.5666738879315));
#18997=CARTESIAN_POINT('',(180.,17.5,-28.5666738879315));
#18998=CARTESIAN_POINT('',(0.,17.5,-28.5666738879315));
#18999=CARTESIAN_POINT('Origin',(0.,20.836901197987,-31.9035750859185));
#19000=CARTESIAN_POINT('',(180.,20.836901197987,-31.9035750859185));
#19001=CARTESIAN_POINT('Origin',(180.,10.4184505989935,0.));
#71773=UNCERTAINTY_MEASURE_WITH_UNIT(LENGTH_MEASURE(0.01),#71796,
'DISTANCE_ACCURACY_VALUE',
'Maximum model space distance between geometric entities at asserted c
onnectivities');
#71783=UNCERTAINTY_MEASURE_WITH_UNIT(LENGTH_MEASURE(0.01),#71796,
'DISTANCE_ACCURACY_VALUE',
'Maximum model space distance between geometric entities at asserted c
onnectivities');
#71785=(
GEOMETRIC_REPRESENTATION_CONTEXT(3)
GLOBAL_UNCERTAINTY_ASSIGNED_CONTEXT((#71773))
GLOBAL_UNIT_ASSIGNED_CONTEXT((#71796,#71798,#71799))
REPRESENTATION_CONTEXT('','3D')
);
#71795=(
GEOMETRIC_REPRESENTATION_CONTEXT(3)
GLOBAL_UNCERTAINTY_ASSIGNED_CONTEXT((#71783))
GLOBAL_UNIT_ASSIGNED_CONTEXT((#71796,#71798,#71799))
REPRESENTATION_CONTEXT('','3D')
);
#71796=(
LENGTH_UNIT()
NAMED_UNIT(*)
SI_UNIT(.MILLI.,.METRE.)
);
#71798=(
NAMED_UNIT(*)
PLANE_ANGLE_UNIT()
SI_UNIT($,.RADIAN.)
);
#71799=(
NAMED_UNIT(*)
SI_UNIT($,.STERADIAN.)
SOLID_ANGLE_UNIT()
);
#71801=SHAPE_DEFINITION_REPRESENTATION(#71812,#72017);
#71812=PRODUCT_DEFINITION_SHAPE('',$,#72029);
#72017=SHAPE_REPRESENTATION('',(#13757),#71785);
#72027=PRODUCT_DEFINITION_CONTEXT('part definition',#72062,'design');
#72029=PRODUCT_DEFINITION('Dual Shaft Rail Support x 180',
'Dual Shaft Rail Support x 180',#72040,#72027);
#72040=PRODUCT_DEFINITION_FORMATION('',$,#72065);
#72062=APPLICATION_CONTEXT(
'Core Data for Automotive Mechanical Design Process');
#72063=PRODUCT_CONTEXT('part definition',#72062,'mechanical');
#72065=PRODUCT('Dual Shaft Rail Support x 180',
'Dual Shaft Rail Support x 180',$,(#72063));
#72076=PRESENTATION_STYLE_ASSIGNMENT((#72087));
#72087=SURFACE_STYLE_USAGE(.BOTH.,#72098);
#72098=SURFACE_SIDE_STYLE('',(#72109));
#72109=SURFACE_STYLE_FILL_AREA(#72120);
#72120=FILL_AREA_STYLE('Opaque(206,210,216)',(#72131));
#72131=FILL_AREA_STYLE_COLOUR('Opaque(206,210,216)',#72142);
#72142=COLOUR_RGB('Opaque(206,210,216)', 0.09019608, 0.27058824, 0.51372549);
ENDSEC;
END-ISO-10303-21;
